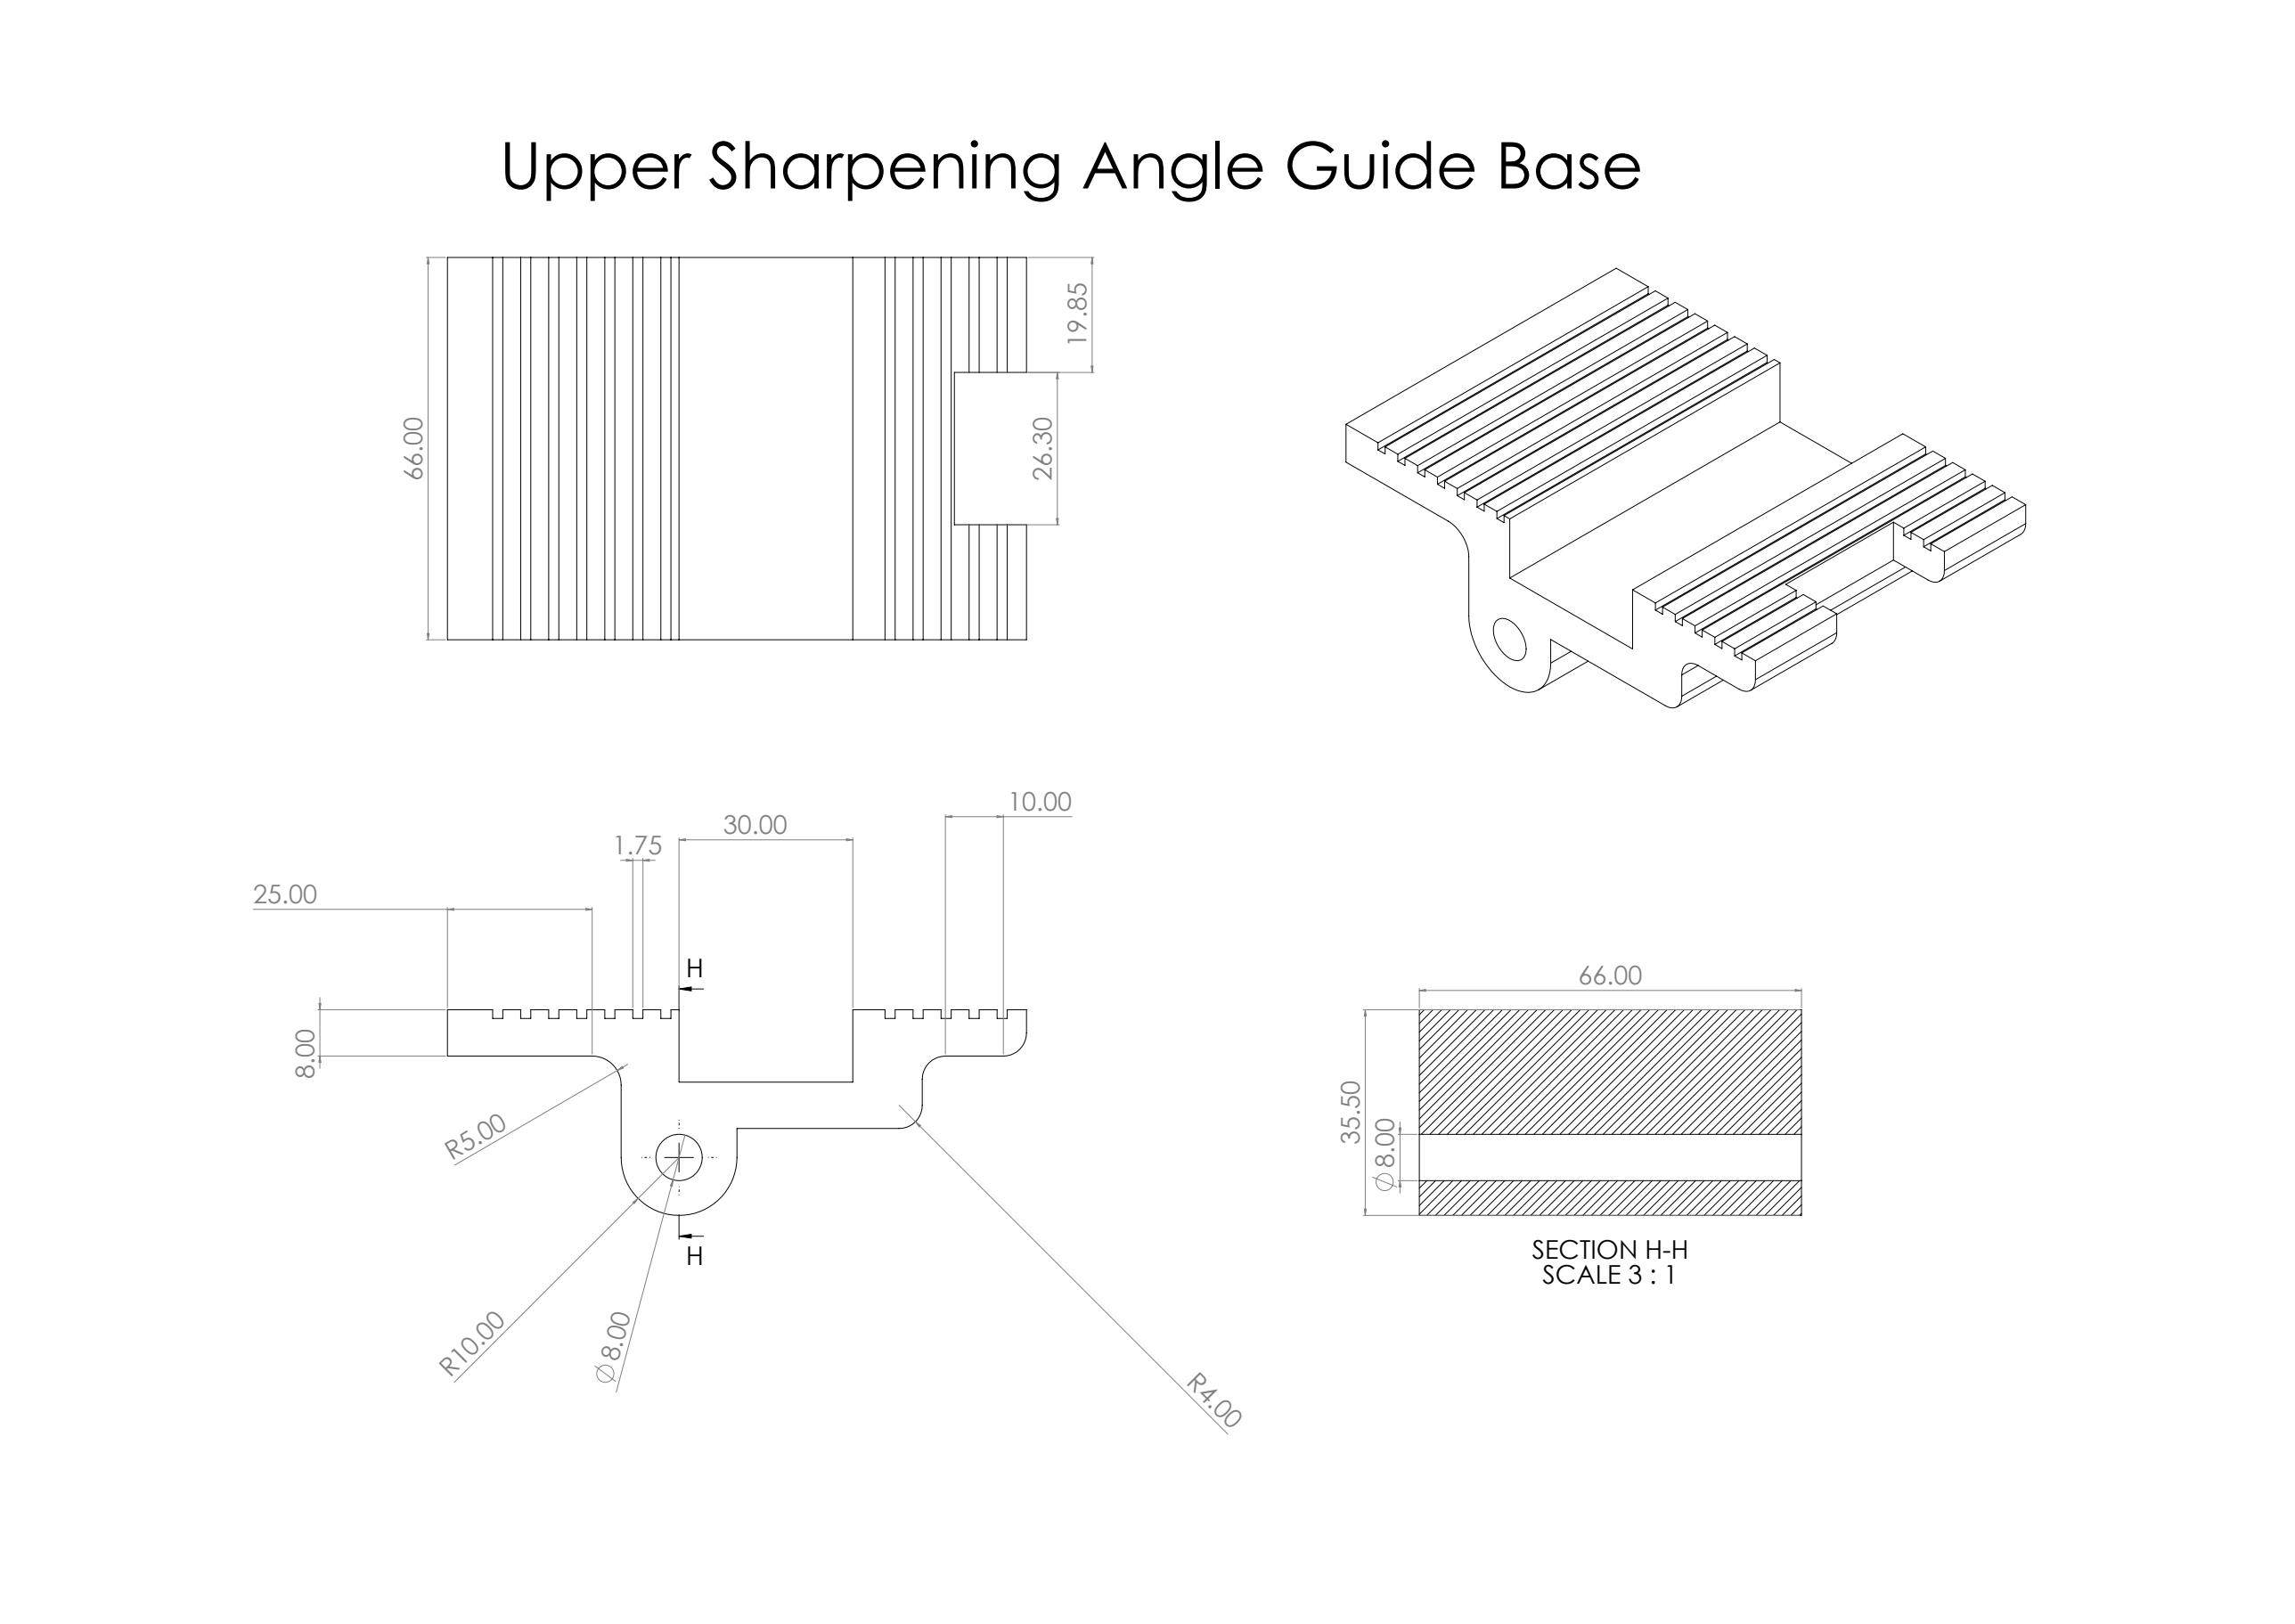
ISO-10303-21;
HEADER;
FILE_DESCRIPTION (('STEP AP214'),
    '1' );
FILE_NAME ('Upper Sharpening Angle Guide Base.step',
    '2026-10-24T21:31:31',
    ( '' ),
    ( '' ),
    'SwSTEP 2.0',
    'SolidWorks 2025',
    '' );
FILE_SCHEMA (( 'AUTOMOTIVE_DESIGN' ));
ENDSEC;

DATA;
#6=LINE ( 'NONE', #11694, #4610 ) ;
#13=LINE ( 'NONE', #7011, #3647 ) ;
#14=VECTOR ( 'NONE', #2004, 1000.000000000000000 ) ;
#17=DIRECTION ( 'NONE',  ( -1.000000000000000000, 0.000000000000000000, 0.000000000000000000 ) ) ;
#20=VERTEX_POINT ( 'NONE', #5429 ) ;
#32=FACE_OUTER_BOUND ( 'NONE', #11110, .T. ) ;
#33=ADVANCED_FACE ( 'NONE', ( #12199 ), #9834, .F. ) ;
#37=ORIENTED_EDGE ( 'NONE', *, *, #2232, .F. ) ;
#38=FACE_OUTER_BOUND ( 'NONE', #6545, .T. ) ;
#41=LINE ( 'NONE', #2497, #6085 ) ;
#42=AXIS2_PLACEMENT_3D ( 'NONE', #10885, #14351, #11948 ) ;
#47=CARTESIAN_POINT ( 'NONE',  ( 46.91810375148135392, 21.75070940071322667, 139.1143251403882459 ) ) ;
#49=CARTESIAN_POINT ( 'NONE',  ( -2.016677571526633510E-15, 23.25070940071368497, -33.00000000000012790 ) ) ;
#54=VECTOR ( 'NONE', #13573, 1000.000000000000000 ) ;
#57=LINE ( 'NONE', #11745, #6919 ) ;
#62=CARTESIAN_POINT ( 'NONE',  ( 114.6731053250840233, 21.75070940071369918, 139.1143251403882459 ) ) ;
#65=VERTEX_POINT ( 'NONE', #11047 ) ;
#66=VECTOR ( 'NONE', #7622, 1000.000000000000000 ) ;
#68=PLANE ( 'NONE',  #7695 ) ;
#72=VERTEX_POINT ( 'NONE', #721 ) ;
#75=PLANE ( 'NONE',  #1648 ) ;
#77=VERTEX_POINT ( 'NONE', #4338 ) ;
#86=VECTOR ( 'NONE', #1332, 1000.000000000000000 ) ;
#94=ORIENTED_EDGE ( 'NONE', *, *, #8937, .F. ) ;
#105=LINE ( 'NONE', #10640, #5976 ) ;
#108=DIRECTION ( 'NONE',  ( 0.000000000000000000, 0.000000000000000000, 1.000000000000000000 ) ) ;
#110=LINE ( 'NONE', #11941, #4147 ) ;
#114=ORIENTED_EDGE ( 'NONE', *, *, #14825, .F. ) ;
#116=CARTESIAN_POINT ( 'NONE',  ( 0.000000000000000000, 21.75070940071363168, 33.00000000000012790 ) ) ;
#118=LINE ( 'NONE', #8565, #1013 ) ;
#120=LINE ( 'NONE', #8431, #11123 ) ;
#130=ORIENTED_EDGE ( 'NONE', *, *, #11606, .T. ) ;
#132=ORIENTED_EDGE ( 'NONE', *, *, #1705, .F. ) ;
#133=DIRECTION ( 'NONE',  ( 1.000000000000000000, 0.000000000000000000, 0.000000000000000000 ) ) ;
#135=ORIENTED_EDGE ( 'NONE', *, *, #2741, .T. ) ;
#138=CARTESIAN_POINT ( 'NONE',  ( 48.00000000000000000, -2.249290599286307479, 139.1143251403882459 ) ) ;
#161=CARTESIAN_POINT ( 'NONE',  ( 42.07846078193830408, 21.75070940071319114, 139.1143251403882459 ) ) ;
#191=DIRECTION ( 'NONE',  ( 0.000000000000000000, 0.000000000000000000, 1.000000000000000000 ) ) ;
#197=DIRECTION ( 'NONE',  ( 1.000000000000000000, 0.000000000000000000, 0.000000000000000000 ) ) ;
#209=ORIENTED_EDGE ( 'NONE', *, *, #14302, .F. ) ;
#216=LINE ( 'NONE', #3742, #12117 ) ;
#218=PLANE ( 'NONE',  #1793 ) ;
#220=ORIENTED_EDGE ( 'NONE', *, *, #12965, .T. ) ;
#221=EDGE_LOOP ( 'NONE', ( #14150, #12830, #6180, #1820 ) ) ;
#222=EDGE_CURVE ( 'NONE', #13907, #15116, #14885, .T. ) ;
#235=LINE ( 'NONE', #14317, #9148 ) ;
#236=CARTESIAN_POINT ( 'NONE',  ( 118.0000000000000568, 2.046973701652633381E-13, 13.14990448602693007 ) ) ;
#240=CARTESIAN_POINT ( 'NONE',  ( 48.00000000000000711, 10.25070940071368497, -33.00000000000012790 ) ) ;
#249=CARTESIAN_POINT ( 'NONE',  ( 104.0000000000000426, 15.25070940071369563, -33.00000000000012790 ) ) ;
#254=FACE_OUTER_BOUND ( 'NONE', #221, .T. ) ;
#255=DIRECTION ( 'NONE',  ( 0.000000000000000000, 0.000000000000000000, -1.000000000000000000 ) ) ;
#257=DIRECTION ( 'NONE',  ( 0.000000000000000000, 1.000000000000000000, -0.000000000000000000 ) ) ;
#265=ORIENTED_EDGE ( 'NONE', *, *, #2651, .T. ) ;
#270=VECTOR ( 'NONE', #1744, 1000.000000000000000 ) ;
#273=DIRECTION ( 'NONE',  ( -0.000000000000000000, -0.000000000000000000, -1.000000000000000000 ) ) ;
#278=DIRECTION ( 'NONE',  ( 0.000000000000000000, 0.000000000000000000, -1.000000000000000000 ) ) ;
#291=VECTOR ( 'NONE', #10970, 1000.000000000000000 ) ;
#299=DIRECTION ( 'NONE',  ( 0.000000000000000000, 1.000000000000000000, 0.000000000000000000 ) ) ;
#315=PLANE ( 'NONE',  #10049 ) ;
#320=VECTOR ( 'NONE', #7998, 1000.000000000000000 ) ;
#321=ORIENTED_EDGE ( 'NONE', *, *, #14732, .T. ) ;
#322=VERTEX_POINT ( 'NONE', #10317 ) ;
#335=EDGE_CURVE ( 'NONE', #11258, #1446, #2933, .T. ) ;
#340=DIRECTION ( 'NONE',  ( 0.000000000000000000, 0.000000000000000000, 1.000000000000000000 ) ) ;
#344=VECTOR ( 'NONE', #582, 1000.000000000000000 ) ;
#351=EDGE_CURVE ( 'NONE', #1115, #11167, #14092, .T. ) ;
#352=CYLINDRICAL_SURFACE ( 'NONE', #8410, 4.000000000000003553 ) ;
#358=VERTEX_POINT ( 'NONE', #2315 ) ;
#359=DIRECTION ( 'NONE',  ( 1.000000000000000000, 0.000000000000000000, 0.000000000000000000 ) ) ;
#360=ORIENTED_EDGE ( 'NONE', *, *, #2072, .T. ) ;
#365=ORIENTED_EDGE ( 'NONE', *, *, #10647, .T. ) ;
#368=CARTESIAN_POINT ( 'NONE',  ( -2.688903428702175252E-15, 23.25070940071368142, 33.00000000000012790 ) ) ;
#370=CARTESIAN_POINT ( 'NONE',  ( 0.000000000000000000, 21.75070940071329417, 139.1143251403882459 ) ) ;
#380=ORIENTED_EDGE ( 'NONE', *, *, #7068, .T. ) ;
#387=EDGE_CURVE ( 'NONE', #550, #2283, #6562, .T. ) ;
#389=ORIENTED_EDGE ( 'NONE', *, *, #387, .F. ) ;
#391=ORIENTED_EDGE ( 'NONE', *, *, #15115, .F. ) ;
#398=CARTESIAN_POINT ( 'NONE',  ( 114.0000000000000284, 15.25070940071369563, 139.1143251403882459 ) ) ;
#402=AXIS2_PLACEMENT_3D ( 'NONE', #1965, #6663, #11352 ) ;
#411=FACE_OUTER_BOUND ( 'NONE', #3533, .T. ) ;
#417=( GEOMETRIC_REPRESENTATION_CONTEXT ( 3 ) GLOBAL_UNCERTAINTY_ASSIGNED_CONTEXT ( ( #1045 ) ) GLOBAL_UNIT_ASSIGNED_CONTEXT ( ( #9181, #13866, #10252 ) ) REPRESENTATION_CONTEXT ( 'NONE', 'WORKASPACE' ) );
#431=EDGE_CURVE ( 'NONE', #7143, #4346, #6, .T. ) ;
#449=EDGE_CURVE ( 'NONE', #4396, #5927, #2469, .T. ) ;
#456=EDGE_LOOP ( 'NONE', ( #15169, #3093, #13253, #6276 ) ) ;
#460=ORIENTED_EDGE ( 'NONE', *, *, #1519, .F. ) ;
#461=DIRECTION ( 'NONE',  ( -0.000000000000000000, -0.000000000000000000, -1.000000000000000000 ) ) ;
#481=PLANE ( 'NONE',  #13025 ) ;
#491=PLANE ( 'NONE',  #9839 ) ;
#514=DIRECTION ( 'NONE',  ( 0.000000000000000000, 1.000000000000000000, -0.000000000000000000 ) ) ;
#525=EDGE_CURVE ( 'NONE', #14965, #13020, #11921, .T. ) ;
#529=ORIENTED_EDGE ( 'NONE', *, *, #4885, .F. ) ;
#535=FACE_OUTER_BOUND ( 'NONE', #14760, .T. ) ;
#537=CARTESIAN_POINT ( 'NONE',  ( 114.6731053250840233, 0.000000000000000000, -33.00000000000012790 ) ) ;
#540=VECTOR ( 'NONE', #9041, 1000.000000000000000 ) ;
#541=CARTESIAN_POINT ( 'NONE',  ( 114.0000000000000284, 19.25070940071369563, 33.00000000000012790 ) ) ;
#542=VECTOR ( 'NONE', #2732, 1000.000000000000000 ) ;
#550=VERTEX_POINT ( 'NONE', #9855 ) ;
#558=AXIS2_PLACEMENT_3D ( 'NONE', #4944, #4869, #3708 ) ;
#560=VECTOR ( 'NONE', #4903, 1000.000000000000000 ) ;
#562=DIRECTION ( 'NONE',  ( -0.000000000000000000, -0.000000000000000000, -1.000000000000000000 ) ) ;
#565=ORIENTED_EDGE ( 'NONE', *, *, #14825, .T. ) ;
#571=LINE ( 'NONE', #6351, #6668 ) ;
#573=ADVANCED_FACE ( 'NONE', ( #1464 ), #315, .F. ) ;
#575=CARTESIAN_POINT ( 'NONE',  ( 95.31453344691183815, 23.25070940071369208, 33.00000000000012790 ) ) ;
#576=ORIENTED_EDGE ( 'NONE', *, *, #10446, .T. ) ;
#577=CARTESIAN_POINT ( 'NONE',  ( 0.000000000000000000, 15.25070940071369563, -13.14990448602693007 ) ) ;
#578=ORIENTED_EDGE ( 'NONE', *, *, #10333, .T. ) ;
#582=DIRECTION ( 'NONE',  ( 0.000000000000000000, 1.000000000000000000, -0.000000000000000000 ) ) ;
#584=ORIENTED_EDGE ( 'NONE', *, *, #12621, .T. ) ;
#587=VERTEX_POINT ( 'NONE', #10936 ) ;
#588=DIRECTION ( 'NONE',  ( -1.000000000000000000, 0.000000000000000000, 0.000000000000000000 ) ) ;
#589=ORIENTED_EDGE ( 'NONE', *, *, #1386, .T. ) ;
#600=CARTESIAN_POINT ( 'NONE',  ( 32.39917484285220439, 21.75070940071312364, 33.00000000000012790 ) ) ;
#613=LINE ( 'NONE', #1772, #10037 ) ;
#620=DIRECTION ( 'NONE',  ( -1.000000000000000000, 0.000000000000000000, 0.000000000000000000 ) ) ;
#626=CARTESIAN_POINT ( 'NONE',  ( 45.17127246049422240, 21.75070940071322667, 139.1143251403882459 ) ) ;
#628=CARTESIAN_POINT ( 'NONE',  ( 43.00000000000000711, 15.25070940071368497, 33.00000000000012790 ) ) ;
#637=CARTESIAN_POINT ( 'NONE',  ( 0.000000000000000000, 15.25070940071369563, 13.14990448602693007 ) ) ;
#642=DIRECTION ( 'NONE',  ( 0.000000000000000000, 0.000000000000000000, 1.000000000000000000 ) ) ;
#647=EDGE_CURVE ( 'NONE', #13534, #13054, #13162, .T. ) ;
#648=LINE ( 'NONE', #5356, #9186 ) ;
#659=CARTESIAN_POINT ( 'NONE',  ( 27.55953187330915810, 23.25070940071368852, -33.00000000000012790 ) ) ;
#660=CARTESIAN_POINT ( 'NONE',  ( 0.000000000000000000, 15.25070940071368497, 139.1143251403882459 ) ) ;
#661=LINE ( 'NONE', #891, #6723 ) ;
#665=VECTOR ( 'NONE', #12241, 1000.000000000000000 ) ;
#675=PRODUCT ( 'Upper Sharpening Angle Guide Base', 'Upper Sharpening Angle Guide Base', '', ( #1396 ) ) ;
#678=ORIENTED_EDGE ( 'NONE', *, *, #2260, .T. ) ;
#686=CARTESIAN_POINT ( 'NONE',  ( 18.00000000000001066, 0.000000000000000000, 139.1143251403882459 ) ) ;
#696=CARTESIAN_POINT ( 'NONE',  ( 25.81270058232203013, 21.75070940071309167, -33.00000000000012790 ) ) ;
#703=AXIS2_PLACEMENT_3D ( 'NONE', #8419, #1403, #8107 ) ;
#719=AXIS2_PLACEMENT_3D ( 'NONE', #5968, #10655, #14038 ) ;
#721=CARTESIAN_POINT ( 'NONE',  ( 114.0000000000000284, 15.25070940071369563, -13.14990448602693007 ) ) ;
#729=ORIENTED_EDGE ( 'NONE', *, *, #11145, .F. ) ;
#731=ORIENTED_EDGE ( 'NONE', *, *, #3102, .F. ) ;
#735=CARTESIAN_POINT ( 'NONE',  ( 68.00000000000001421, -2.249290599286293268, 33.00000000000012790 ) ) ;
#738=DIRECTION ( 'NONE',  ( 1.110223024625156540E-15, -1.000000000000000000, 0.000000000000000000 ) ) ;
#741=ADVANCED_FACE ( 'NONE', ( #11639 ), #15109, .F. ) ;
#745=ORIENTED_EDGE ( 'NONE', *, *, #13734, .T. ) ;
#749=ORIENTED_EDGE ( 'NONE', *, *, #11198, .T. ) ;
#751=ADVANCED_FACE ( 'NONE', ( #11790, #1325 ), #12724, .F. ) ;
#757=DIRECTION ( 'NONE',  ( -2.775557561562891351E-15, 1.000000000000000000, 0.000000000000000000 ) ) ;
#766=ORIENTED_EDGE ( 'NONE', *, *, #5761, .T. ) ;
#767=VECTOR ( 'NONE', #133, 1000.000000000000000 ) ;
#778=CARTESIAN_POINT ( 'NONE',  ( 118.0000000000000284, 23.25070940071369563, 139.1143251403882459 ) ) ;
#782=CARTESIAN_POINT ( 'NONE',  ( 30.65234355186507997, 21.75070940071312364, 139.1143251403882459 ) ) ;
#794=ORIENTED_EDGE ( 'NONE', *, *, #3873, .F. ) ;
#799=ADVANCED_FACE ( 'NONE', ( #1173 ), #14109, .F. ) ;
#804=CARTESIAN_POINT ( 'NONE',  ( 51.75774672102440377, 21.75070940071325865, -33.00000000000012790 ) ) ;
#809=ORIENTED_EDGE ( 'NONE', *, *, #5886, .F. ) ;
#812=CARTESIAN_POINT ( 'NONE',  ( 103.2469880950108063, 23.25070940071369208, -33.00000000000012790 ) ) ;
#813=LINE ( 'NONE', #2986, #1383 ) ;
#815=CARTESIAN_POINT ( 'NONE',  ( 46.91810375148135392, 23.25070940071368852, 33.00000000000012790 ) ) ;
#826=ORIENTED_EDGE ( 'NONE', *, *, #11805, .F. ) ;
#830=CARTESIAN_POINT ( 'NONE',  ( 100.0000000000000284, 11.25070940071369563, -33.00000000000012790 ) ) ;
#836=FACE_OUTER_BOUND ( 'NONE', #10102, .T. ) ;
#837=ADVANCED_FACE ( 'NONE', ( #8103 ), #14260, .F. ) ;
#838=ORIENTED_EDGE ( 'NONE', *, *, #12621, .F. ) ;
#844=VERTEX_POINT ( 'NONE', #5167 ) ;
#845=ADVANCED_FACE ( 'NONE', ( #1698 ), #6393, .F. ) ;
#847=LINE ( 'NONE', #1850, #4677 ) ;
#850=DIRECTION ( 'NONE',  ( 1.000000000000000000, 1.156482317317870492E-16, 0.000000000000000000 ) ) ;
#855=LINE ( 'NONE', #14787, #8320 ) ;
#857=APPLICATION_CONTEXT ( 'automotive_design' ) ;
#862=FACE_OUTER_BOUND ( 'NONE', #2285, .T. ) ;
#868=ORIENTED_EDGE ( 'NONE', *, *, #13611, .F. ) ;
#869=CARTESIAN_POINT ( 'NONE',  ( 30.65234355186507997, 23.25070940071368852, 33.00000000000012790 ) ) ;
#871=ORIENTED_EDGE ( 'NONE', *, *, #15074, .F. ) ;
#874=AXIS2_PLACEMENT_3D ( 'NONE', #14984, #10447, #6820 ) ;
#891=CARTESIAN_POINT ( 'NONE',  ( -2.016677571526633510E-15, 23.25070940071368497, 33.00000000000012790 ) ) ;
#906=EDGE_LOOP ( 'NONE', ( #132, #13235, #5815, #2969 ) ) ;
#914=CARTESIAN_POINT ( 'NONE',  ( 109.8334623555409735, 0.000000000000000000, 13.14990448602693007 ) ) ;
#916=VECTOR ( 'NONE', #1039, 1000.000000000000000 ) ;
#925=DIRECTION ( 'NONE',  ( 0.000000000000000000, 1.000000000000000000, 0.000000000000000000 ) ) ;
#930=CARTESIAN_POINT ( 'NONE',  ( 112.9262740340969060, 0.000000000000000000, 139.1143251403882459 ) ) ;
#937=EDGE_CURVE ( 'NONE', #7143, #11623, #10072, .T. ) ;
#941=CARTESIAN_POINT ( 'NONE',  ( 0.000000000000000000, 21.75070940071325865, 139.1143251403882459 ) ) ;
#957=CARTESIAN_POINT ( 'NONE',  ( 40.33162949095117966, 23.25070940071368852, -33.00000000000012790 ) ) ;
#970=AXIS2_PLACEMENT_3D ( 'NONE', #941, #13800, #11326 ) ;
#973=DIRECTION ( 'NONE',  ( 1.000000000000000000, 1.156482317317870492E-16, 0.000000000000000000 ) ) ;
#977=VERTEX_POINT ( 'NONE', #14993 ) ;
#980=CARTESIAN_POINT ( 'NONE',  ( -2.688903428702175252E-15, 23.25070940071368142, 33.00000000000012790 ) ) ;
#982=AXIS2_PLACEMENT_3D ( 'NONE', #8563, #2856, #340 ) ;
#992=CARTESIAN_POINT ( 'NONE',  ( 0.000000000000000000, 21.75070940071309167, 139.1143251403882459 ) ) ;
#1003=ORIENTED_EDGE ( 'NONE', *, *, #8126, .F. ) ;
#1007=DIRECTION ( 'NONE',  ( -0.000000000000000000, -0.000000000000000000, -1.000000000000000000 ) ) ;
#1012=DIRECTION ( 'NONE',  ( -0.000000000000000000, 0.000000000000000000, 1.000000000000000000 ) ) ;
#1013=VECTOR ( 'NONE', #13265, 1000.000000000000000 ) ;
#1035=LINE ( 'NONE', #2428, #12248 ) ;
#1037=CARTESIAN_POINT ( 'NONE',  ( 27.55953187330915810, 21.75070940071309167, 139.1143251403882459 ) ) ;
#1039=DIRECTION ( 'NONE',  ( -1.000000000000000000, -1.156482317317870492E-16, 0.000000000000000000 ) ) ;
#1045=UNCERTAINTY_MEASURE_WITH_UNIT (LENGTH_MEASURE( 1.000000000000000082E-05 ), #9181, 'distance_accuracy_value', 'NONE');
#1047=ORIENTED_EDGE ( 'NONE', *, *, #11121, .T. ) ;
#1053=ADVANCED_FACE ( 'NONE', ( #1060 ), #68, .F. ) ;
#1054=CARTESIAN_POINT ( 'NONE',  ( 45.17127246049422240, 21.75070940071322667, 33.00000000000012790 ) ) ;
#1060=FACE_OUTER_BOUND ( 'NONE', #4938, .T. ) ;
#1074=DIRECTION ( 'NONE',  ( 0.000000000000000000, 1.000000000000000000, -0.000000000000000000 ) ) ;
#1091=CARTESIAN_POINT ( 'NONE',  ( -2.688903428702175252E-15, 23.25070940071368142, 139.1143251403882459 ) ) ;
#1104=DIRECTION ( 'NONE',  ( 0.000000000000000000, 1.000000000000000000, 0.000000000000000000 ) ) ;
#1110=LINE ( 'NONE', #2350, #5012 ) ;
#1115=VERTEX_POINT ( 'NONE', #10454 ) ;
#1117=VERTEX_POINT ( 'NONE', #9537 ) ;
#1120=DIRECTION ( 'NONE',  ( -1.000000000000000000, 0.000000000000000000, 0.000000000000000000 ) ) ;
#1121=VECTOR ( 'NONE', #11160, 1000.000000000000000 ) ;
#1127=CARTESIAN_POINT ( 'NONE',  ( 50.01091543003727224, 0.000000000000000000, -33.00000000000012790 ) ) ;
#1132=ORIENTED_EDGE ( 'NONE', *, *, #2690, .T. ) ;
#1137=ORIENTED_EDGE ( 'NONE', *, *, #10778, .F. ) ;
#1143=EDGE_CURVE ( 'NONE', #6567, #14796, #12851, .T. ) ;
#1144=AXIS2_PLACEMENT_3D ( 'NONE', #660, #5528, #12372 ) ;
#1146=DIRECTION ( 'NONE',  ( 1.000000000000000000, -0.000000000000000000, -0.000000000000000000 ) ) ;
#1150=DIRECTION ( 'NONE',  ( 1.734723475976807292E-15, -1.000000000000000000, 0.000000000000000000 ) ) ;
#1151=CARTESIAN_POINT ( 'NONE',  ( 54.00000000000000711, -2.249290599286311032, 33.00000000000012790 ) ) ;
#1153=ADVANCED_FACE ( 'NONE', ( #11515 ), #2215, .F. ) ;
#1173=FACE_OUTER_BOUND ( 'NONE', #9518, .T. ) ;
#1175=EDGE_CURVE ( 'NONE', #10461, #3922, #7367, .T. ) ;
#1176=VECTOR ( 'NONE', #14022, 1000.000000000000000 ) ;
#1178=FACE_OUTER_BOUND ( 'NONE', #3126, .T. ) ;
#1189=VECTOR ( 'NONE', #10286, 1000.000000000000000 ) ;
#1190=EDGE_LOOP ( 'NONE', ( #8131, #3911, #5540, #4860 ) ) ;
#1205=ORIENTED_EDGE ( 'NONE', *, *, #6548, .T. ) ;
#1216=ORIENTED_EDGE ( 'NONE', *, *, #4415, .T. ) ;
#1222=EDGE_CURVE ( 'NONE', #20, #13907, #11903, .T. ) ;
#1225=EDGE_LOOP ( 'NONE', ( #8488, #1205, #7597, #4474 ) ) ;
#1231=DIRECTION ( 'NONE',  ( 1.000000000000000000, 0.000000000000000000, 0.000000000000000000 ) ) ;
#1239=DIRECTION ( 'NONE',  ( -1.110223024625156540E-15, 1.000000000000000000, 0.000000000000000000 ) ) ;
#1254=VECTOR ( 'NONE', #14887, 1000.000000000000000 ) ;
#1256=ORIENTED_EDGE ( 'NONE', *, *, #1813, .F. ) ;
#1257=DIRECTION ( 'NONE',  ( 0.000000000000000000, 0.000000000000000000, 1.000000000000000000 ) ) ;
#1261=ADVANCED_FACE ( 'NONE', ( #9762 ), #6148, .T. ) ;
#1262=CARTESIAN_POINT ( 'NONE',  ( -1.243300532054838308E-15, 10.75070940071368142, -33.00000000000012790 ) ) ;
#1263=VECTOR ( 'NONE', #5764, 1000.000000000000000 ) ;
#1275=LINE ( 'NONE', #10675, #767 ) ;
#1280=ADVANCED_FACE ( 'NONE', ( #8522, #10758 ), #218, .T. ) ;
#1288=AXIS2_PLACEMENT_3D ( 'NONE', #12935, #13082, #1377 ) ;
#1289=EDGE_LOOP ( 'NONE', ( #2796, #13787, #11153, #13533, #11758, #578, #321, #745 ) ) ;
#1297=VECTOR ( 'NONE', #3657, 1000.000000000000000 ) ;
#1300=CARTESIAN_POINT ( 'NONE',  ( -2.688903428702175252E-15, 23.25070940071368142, 33.00000000000012790 ) ) ;
#1308=DIRECTION ( 'NONE',  ( -0.000000000000000000, -0.000000000000000000, -1.000000000000000000 ) ) ;
#1312=VECTOR ( 'NONE', #7448, 1000.000000000000000 ) ;
#1324=LINE ( 'NONE', #11711, #12676 ) ;
#1325=FACE_BOUND ( 'NONE', #10555, .T. ) ;
#1332=DIRECTION ( 'NONE',  ( -1.000000000000000000, -8.673617379884035472E-17, 0.000000000000000000 ) ) ;
#1346=EDGE_CURVE ( 'NONE', #358, #13613, #648, .T. ) ;
#1352=DIRECTION ( 'NONE',  ( 0.000000000000000000, 1.000000000000000000, -0.000000000000000000 ) ) ;
#1355=DIRECTION ( 'NONE',  ( 0.000000000000000000, 1.000000000000000000, -0.000000000000000000 ) ) ;
#1361=EDGE_CURVE ( 'NONE', #6460, #12669, #7742, .T. ) ;
#1364=EDGE_CURVE ( 'NONE', #11647, #12323, #3195, .T. ) ;
#1367=ORIENTED_EDGE ( 'NONE', *, *, #15114, .T. ) ;
#1377=DIRECTION ( 'NONE',  ( 0.000000000000000000, 0.000000000000000000, 1.000000000000000000 ) ) ;
#1379=DIRECTION ( 'NONE',  ( 0.000000000000000000, -1.000000000000000000, 0.000000000000000000 ) ) ;
#1381=EDGE_LOOP ( 'NONE', ( #15083, #10267, #135, #6493 ) ) ;
#1382=EDGE_CURVE ( 'NONE', #13652, #4131, #6504, .T. ) ;
#1383=VECTOR ( 'NONE', #1822, 1000.000000000000000 ) ;
#1385=LINE ( 'NONE', #5078, #7650 ) ;
#1386=EDGE_CURVE ( 'NONE', #5719, #5462, #7705, .T. ) ;
#1391=ORIENTED_EDGE ( 'NONE', *, *, #13173, .T. ) ;
#1394=ORIENTED_EDGE ( 'NONE', *, *, #6976, .F. ) ;
#1396=PRODUCT_CONTEXT ( 'NONE', #857, 'mechanical' ) ;
#1397=DIRECTION ( 'NONE',  ( 1.000000000000000000, 1.156482317317870492E-16, 0.000000000000000000 ) ) ;
#1398=DIRECTION ( 'NONE',  ( 0.000000000000000000, 1.000000000000000000, -0.000000000000000000 ) ) ;
#1401=VECTOR ( 'NONE', #6292, 1000.000000000000000 ) ;
#1403=DIRECTION ( 'NONE',  ( 0.000000000000000000, 0.000000000000000000, -1.000000000000000000 ) ) ;
#1414=CARTESIAN_POINT ( 'NONE',  ( 35.49198652140812982, 23.25070940071368852, -33.00000000000012790 ) ) ;
#1426=ORIENTED_EDGE ( 'NONE', *, *, #10139, .F. ) ;
#1438=CARTESIAN_POINT ( 'NONE',  ( 58.00000000000000711, 0.000000000000000000, 33.00000000000012790 ) ) ;
#1444=LINE ( 'NONE', #4764, #6559 ) ;
#1445=ORIENTED_EDGE ( 'NONE', *, *, #12870, .T. ) ;
#1446=VERTEX_POINT ( 'NONE', #7822 ) ;
#1448=ORIENTED_EDGE ( 'NONE', *, *, #8487, .F. ) ;
#1457=EDGE_CURVE ( 'NONE', #3968, #9234, #11416, .T. ) ;
#1460=VERTEX_POINT ( 'NONE', #804 ) ;
#1464=FACE_OUTER_BOUND ( 'NONE', #14437, .T. ) ;
#1467=ORIENTED_EDGE ( 'NONE', *, *, #4385, .F. ) ;
#1472=CARTESIAN_POINT ( 'NONE',  ( 54.85055839958032209, 21.75070940071329417, -33.00000000000012790 ) ) ;
#1501=AXIS2_PLACEMENT_3D ( 'NONE', #5150, #14538, #4054 ) ;
#1506=VERTEX_POINT ( 'NONE', #8049 ) ;
#1510=AXIS2_PLACEMENT_3D ( 'NONE', #4667, #12835, #13133 ) ;
#1511=CARTESIAN_POINT ( 'NONE',  ( 35.49198652140812982, 21.75070940071315562, -33.00000000000012790 ) ) ;
#1519=EDGE_CURVE ( 'NONE', #14965, #977, #1110, .T. ) ;
#1524=EDGE_LOOP ( 'NONE', ( #11746, #12539, #5464, #7230 ) ) ;
#1527=VERTEX_POINT ( 'NONE', #957 ) ;
#1529=EDGE_CURVE ( 'NONE', #4620, #12466, #3431, .T. ) ;
#1537=ORIENTED_EDGE ( 'NONE', *, *, #6853, .F. ) ;
#1549=VERTEX_POINT ( 'NONE', #10515 ) ;
#1551=VECTOR ( 'NONE', #10800, 1000.000000000000000 ) ;
#1555=CARTESIAN_POINT ( 'NONE',  ( 0.000000000000000000, 21.75070940071369918, -33.00000000000012790 ) ) ;
#1556=LINE ( 'NONE', #5543, #8188 ) ;
#1559=ORIENTED_EDGE ( 'NONE', *, *, #10247, .T. ) ;
#1567=EDGE_CURVE ( 'NONE', #3404, #4646, #2275, .T. ) ;
#1570=CARTESIAN_POINT ( 'NONE',  ( 30.65234355186507997, 21.75070940071312364, -33.00000000000012790 ) ) ;
#1581=CARTESIAN_POINT ( 'NONE',  ( 112.9262740340969060, 0.000000000000000000, -33.00000000000012790 ) ) ;
#1583=CARTESIAN_POINT ( 'NONE',  ( 18.00000000000001066, 0.000000000000000000, -33.00000000000012790 ) ) ;
#1593=CARTESIAN_POINT ( 'NONE',  ( 112.9262740340969060, 0.000000000000000000, 33.00000000000012790 ) ) ;
#1614=CARTESIAN_POINT ( 'NONE',  ( 114.6731053250840233, 23.25070940071369563, 139.1143251403882459 ) ) ;
#1629=DIRECTION ( 'NONE',  ( -0.000000000000000000, -0.000000000000000000, 1.000000000000000000 ) ) ;
#1632=VECTOR ( 'NONE', #13443, 1000.000000000000000 ) ;
#1648=AXIS2_PLACEMENT_3D ( 'NONE', #11908, #9701, #13294 ) ;
#1650=DIRECTION ( 'NONE',  ( 0.000000000000000000, 1.000000000000000000, -0.000000000000000000 ) ) ;
#1670=DIRECTION ( 'NONE',  ( 0.000000000000000000, 1.000000000000000000, -0.000000000000000000 ) ) ;
#1672=ORIENTED_EDGE ( 'NONE', *, *, #10963, .F. ) ;
#1674=ORIENTED_EDGE ( 'NONE', *, *, #3328, .F. ) ;
#1679=VERTEX_POINT ( 'NONE', #8025 ) ;
#1682=CARTESIAN_POINT ( 'NONE',  ( 105.5545870572953930, 15.25070940071369563, -13.14990448602692474 ) ) ;
#1691=VERTEX_POINT ( 'NONE', #3410 ) ;
#1692=ORIENTED_EDGE ( 'NONE', *, *, #11765, .T. ) ;
#1697=DIRECTION ( 'NONE',  ( 0.000000000000000000, 1.000000000000000000, -0.000000000000000000 ) ) ;
#1698=FACE_OUTER_BOUND ( 'NONE', #8312, .T. ) ;
#1705=EDGE_CURVE ( 'NONE', #20, #9290, #6865, .T. ) ;
#1707=FACE_OUTER_BOUND ( 'NONE', #14370, .T. ) ;
#1721=EDGE_CURVE ( 'NONE', #13543, #1911, #5496, .T. ) ;
#1733=DIRECTION ( 'NONE',  ( -0.000000000000000000, -0.000000000000000000, -1.000000000000000000 ) ) ;
#1744=DIRECTION ( 'NONE',  ( 0.000000000000000000, 1.000000000000000000, -0.000000000000000000 ) ) ;
#1757=DIRECTION ( 'NONE',  ( -0.000000000000000000, -0.000000000000000000, -1.000000000000000000 ) ) ;
#1760=FACE_OUTER_BOUND ( 'NONE', #8836, .T. ) ;
#1772=CARTESIAN_POINT ( 'NONE',  ( 54.00000000000000711, -2.249290599286311032, 139.1143251403882459 ) ) ;
#1773=AXIS2_PLACEMENT_3D ( 'NONE', #8136, #7618, #11156 ) ;
#1779=ORIENTED_EDGE ( 'NONE', *, *, #6089, .F. ) ;
#1788=VERTEX_POINT ( 'NONE', #8494 ) ;
#1790=EDGE_CURVE ( 'NONE', #8955, #2597, #4873, .T. ) ;
#1793=AXIS2_PLACEMENT_3D ( 'NONE', #6361, #13067, #12201 ) ;
#1807=LINE ( 'NONE', #637, #3513 ) ;
#1809=VERTEX_POINT ( 'NONE', #4945 ) ;
#1813=EDGE_CURVE ( 'NONE', #9234, #13543, #6111, .T. ) ;
#1820=ORIENTED_EDGE ( 'NONE', *, *, #3813, .F. ) ;
#1822=DIRECTION ( 'NONE',  ( -0.000000000000000000, -0.000000000000000000, -1.000000000000000000 ) ) ;
#1830=ADVANCED_FACE ( 'NONE', ( #8267 ), #6033, .T. ) ;
#1833=DIRECTION ( 'NONE',  ( 0.000000000000000000, 1.000000000000000000, -0.000000000000000000 ) ) ;
#1834=VERTEX_POINT ( 'NONE', #9654 ) ;
#1838=VERTEX_POINT ( 'NONE', #13180 ) ;
#1841=ADVANCED_FACE ( 'NONE', ( #1178 ), #14413, .T. ) ;
#1844=VERTEX_POINT ( 'NONE', #10571 ) ;
#1846=CARTESIAN_POINT ( 'NONE',  ( 45.17127246049422240, 0.000000000000000000, 33.00000000000012790 ) ) ;
#1848=ORIENTED_EDGE ( 'NONE', *, *, #2501, .F. ) ;
#1850=CARTESIAN_POINT ( 'NONE',  ( 95.31453344691183815, 23.25070940071369208, 139.1143251403882459 ) ) ;
#1860=PLANE ( 'NONE',  #8128 ) ;
#1866=DIRECTION ( 'NONE',  ( 1.156482317317871725E-16, -1.000000000000000000, 0.000000000000000000 ) ) ;
#1872=EDGE_CURVE ( 'NONE', #1691, #14241, #5960, .T. ) ;
#1883=EDGE_CURVE ( 'NONE', #7515, #2307, #5845, .T. ) ;
#1893=CARTESIAN_POINT ( 'NONE',  ( 35.49198652140812982, 0.000000000000000000, 139.1143251403882459 ) ) ;
#1905=VERTEX_POINT ( 'NONE', #3048 ) ;
#1907=VERTEX_POINT ( 'NONE', #7892 ) ;
#1908=CARTESIAN_POINT ( 'NONE',  ( 42.07846078193830408, 23.25070940071368852, -33.00000000000012790 ) ) ;
#1911=VERTEX_POINT ( 'NONE', #4339 ) ;
#1920=DIRECTION ( 'NONE',  ( -2.775557561562891351E-15, 1.000000000000000000, 0.000000000000000000 ) ) ;
#1924=ORIENTED_EDGE ( 'NONE', *, *, #3689, .F. ) ;
#1926=CARTESIAN_POINT ( 'NONE',  ( 54.85055839958032209, 0.000000000000000000, 139.1143251403882459 ) ) ;
#1927=ORIENTED_EDGE ( 'NONE', *, *, #12887, .F. ) ;
#1932=CARTESIAN_POINT ( 'NONE',  ( 112.9262740340969060, 23.25070940071369563, 139.1143251403882459 ) ) ;
#1938=AXIS2_PLACEMENT_3D ( 'NONE', #13715, #5489, #850 ) ;
#1948=DIRECTION ( 'NONE',  ( -1.000000000000000000, 0.000000000000000000, 0.000000000000000000 ) ) ;
#1956=DIRECTION ( 'NONE',  ( 0.000000000000000000, -1.000000000000000000, 0.000000000000000000 ) ) ;
#1958=VECTOR ( 'NONE', #6701, 1000.000000000000000 ) ;
#1965=CARTESIAN_POINT ( 'NONE',  ( 51.75774672102440377, 0.000000000000000000, 139.1143251403882459 ) ) ;
#1972=ORIENTED_EDGE ( 'NONE', *, *, #7774, .T. ) ;
#1983=CARTESIAN_POINT ( 'NONE',  ( 98.40734512546775647, 23.25070940071369208, -33.00000000000012790 ) ) ;
#1996=CARTESIAN_POINT ( 'NONE',  ( 108.0866310645538562, 23.25070940071369563, 33.00000000000012790 ) ) ;
#2004=DIRECTION ( 'NONE',  ( 0.000000000000000000, 1.000000000000000000, -0.000000000000000000 ) ) ;
#2005=EDGE_LOOP ( 'NONE', ( #13844, #10093, #5618, #6415 ) ) ;
#2009=FACE_OUTER_BOUND ( 'NONE', #13278, .T. ) ;
#2019=EDGE_CURVE ( 'NONE', #8234, #7396, #8440, .T. ) ;
#2029=LINE ( 'NONE', #6722, #8175 ) ;
#2031=CARTESIAN_POINT ( 'NONE',  ( 50.01091543003727224, 0.000000000000000000, 33.00000000000012790 ) ) ;
#2042=VECTOR ( 'NONE', #13527, 1000.000000000000000 ) ;
#2044=DIRECTION ( 'NONE',  ( 0.000000000000000000, 0.000000000000000000, -1.000000000000000000 ) ) ;
#2045=AXIS2_PLACEMENT_3D ( 'NONE', #2916, #4283, #8985 ) ;
#2055=ORIENTED_EDGE ( 'NONE', *, *, #13611, .T. ) ;
#2066=LINE ( 'NONE', #14079, #8795 ) ;
#2072=EDGE_CURVE ( 'NONE', #844, #13652, #11497, .T. ) ;
#2073=CARTESIAN_POINT ( 'NONE',  ( 114.6731053250840233, 21.75070940071369918, 139.1143251403882459 ) ) ;
#2083=EDGE_CURVE ( 'NONE', #12669, #3922, #4810, .T. ) ;
#2084=LINE ( 'NONE', #12556, #14 ) ;
#2086=CARTESIAN_POINT ( 'NONE',  ( 130.4454129427046496, 23.25070940071369563, -13.14990448602692474 ) ) ;
#2090=ORIENTED_EDGE ( 'NONE', *, *, #525, .T. ) ;
#2096=ORIENTED_EDGE ( 'NONE', *, *, #9756, .F. ) ;
#2097=ORIENTED_EDGE ( 'NONE', *, *, #7253, .F. ) ;
#2099=CARTESIAN_POINT ( 'NONE',  ( 112.9262740340969060, 21.75070940071369918, 33.00000000000012790 ) ) ;
#2117=EDGE_LOOP ( 'NONE', ( #3377, #9705, #678, #7452 ) ) ;
#2119=VECTOR ( 'NONE', #2226, 1000.000000000000000 ) ;
#2120=ORIENTED_EDGE ( 'NONE', *, *, #8390, .T. ) ;
#2122=VECTOR ( 'NONE', #7507, 1000.000000000000000 ) ;
#2123=EDGE_CURVE ( 'NONE', #8184, #7261, #9511, .T. ) ;
#2124=FACE_OUTER_BOUND ( 'NONE', #9570, .T. ) ;
#2134=CARTESIAN_POINT ( 'NONE',  ( 62.00000000000001421, -2.249290599286310588, 139.1143251403882459 ) ) ;
#2144=EDGE_CURVE ( 'NONE', #1115, #5061, #1035, .T. ) ;
#2148=DIRECTION ( 'NONE',  ( -0.000000000000000000, -0.000000000000000000, -1.000000000000000000 ) ) ;
#2149=CARTESIAN_POINT ( 'NONE',  ( 103.2469880950108063, 23.25070940071369208, 33.00000000000012790 ) ) ;
#2150=ORIENTED_EDGE ( 'NONE', *, *, #3689, .T. ) ;
#2157=AXIS2_PLACEMENT_3D ( 'NONE', #2634, #7329, #9578 ) ;
#2165=DIRECTION ( 'NONE',  ( 0.000000000000000000, -0.000000000000000000, 1.000000000000000000 ) ) ;
#2167=EDGE_LOOP ( 'NONE', ( #2376, #14738, #11687, #7222 ) ) ;
#2174=EDGE_CURVE ( 'NONE', #8402, #322, #15127, .T. ) ;
#2178=DIRECTION ( 'NONE',  ( -0.000000000000000000, -0.000000000000000000, -1.000000000000000000 ) ) ;
#2189=ORIENTED_EDGE ( 'NONE', *, *, #8041, .T. ) ;
#2191=CARTESIAN_POINT ( 'NONE',  ( 37.23881781239525424, 21.75070940071315562, 139.1143251403882459 ) ) ;
#2197=CARTESIAN_POINT ( 'NONE',  ( 105.5545870572953930, -1.749290599286305259, 13.14990448602692474 ) ) ;
#2201=ORIENTED_EDGE ( 'NONE', *, *, #14114, .F. ) ;
#2203=ORIENTED_EDGE ( 'NONE', *, *, #9582, .F. ) ;
#2210=PLANE ( 'NONE',  #874 ) ;
#2215=PLANE ( 'NONE',  #10403 ) ;
#2216=ADVANCED_FACE ( 'NONE', ( #13199 ), #4069, .F. ) ;
#2226=DIRECTION ( 'NONE',  ( -1.000000000000000000, -1.156482317317870492E-16, 0.000000000000000000 ) ) ;
#2227=PLANE ( 'NONE',  #7931 ) ;
#2231=ORIENTED_EDGE ( 'NONE', *, *, #2415, .T. ) ;
#2232=EDGE_CURVE ( 'NONE', #2283, #1907, #613, .T. ) ;
#2236=CARTESIAN_POINT ( 'NONE',  ( 48.00000000000000000, -2.664535259100377906E-14, 33.00000000000012790 ) ) ;
#2241=DIRECTION ( 'NONE',  ( -5.551115123125787632E-16, -1.000000000000000000, 0.000000000000000000 ) ) ;
#2252=CARTESIAN_POINT ( 'NONE',  ( 35.49198652140812982, 23.25070940071368852, 33.00000000000012790 ) ) ;
#2259=ORIENTED_EDGE ( 'NONE', *, *, #3210, .F. ) ;
#2260=EDGE_CURVE ( 'NONE', #8536, #12694, #13705, .T. ) ;
#2261=CARTESIAN_POINT ( 'NONE',  ( -2.688903428702175252E-15, 23.25070940071368142, 139.1143251403882459 ) ) ;
#2265=AXIS2_PLACEMENT_3D ( 'NONE', #9325, #11542, #1239 ) ;
#2273=DIRECTION ( 'NONE',  ( -0.000000000000000000, -0.000000000000000000, -1.000000000000000000 ) ) ;
#2275=LINE ( 'NONE', #49, #1189 ) ;
#2283=VERTEX_POINT ( 'NONE', #1151 ) ;
#2285=EDGE_LOOP ( 'NONE', ( #11883, #9864, #9691, #10059 ) ) ;
#2287=ADVANCED_FACE ( 'NONE', ( #15012 ), #11382, .T. ) ;
#2294=ORIENTED_EDGE ( 'NONE', *, *, #1364, .F. ) ;
#2307=VERTEX_POINT ( 'NONE', #15093 ) ;
#2312=LINE ( 'NONE', #11690, #8406 ) ;
#2314=VERTEX_POINT ( 'NONE', #4542 ) ;
#2315=CARTESIAN_POINT ( 'NONE',  ( 118.0000000000000284, 23.25070940071369563, 33.00000000000012790 ) ) ;
#2326=CARTESIAN_POINT ( 'NONE',  ( 109.8334623555409735, 23.25070940071369563, 139.1143251403882459 ) ) ;
#2327=DIRECTION ( 'NONE',  ( 0.000000000000000000, 0.000000000000000000, 1.000000000000000000 ) ) ;
#2328=ORIENTED_EDGE ( 'NONE', *, *, #13643, .T. ) ;
#2335=DIRECTION ( 'NONE',  ( -1.000000000000000000, 0.000000000000000000, 0.000000000000000000 ) ) ;
#2350=CARTESIAN_POINT ( 'NONE',  ( -2.016677571526633510E-15, 23.25070940071368497, 33.00000000000012790 ) ) ;
#2352=ADVANCED_FACE ( 'NONE', ( #4623 ), #3158, .T. ) ;
#2356=ORIENTED_EDGE ( 'NONE', *, *, #6494, .T. ) ;
#2358=CARTESIAN_POINT ( 'NONE',  ( 118.0000000000000284, 23.25070940071369563, 13.14990448602692474 ) ) ;
#2365=LINE ( 'NONE', #138, #12596 ) ;
#2376=ORIENTED_EDGE ( 'NONE', *, *, #12041, .F. ) ;
#2392=AXIS2_PLACEMENT_3D ( 'NONE', #11950, #4573, #7115 ) ;
#2398=ORIENTED_EDGE ( 'NONE', *, *, #937, .F. ) ;
#2405=VECTOR ( 'NONE', #14297, 1000.000000000000000 ) ;
#2408=AXIS2_PLACEMENT_3D ( 'NONE', #6503, #11193, #642 ) ;
#2415=EDGE_CURVE ( 'NONE', #587, #13534, #7090, .T. ) ;
#2422=DIRECTION ( 'NONE',  ( -0.000000000000000000, -0.000000000000000000, -1.000000000000000000 ) ) ;
#2423=AXIS2_PLACEMENT_3D ( 'NONE', #10552, #13856, #9169 ) ;
#2424=ORIENTED_EDGE ( 'NONE', *, *, #1386, .F. ) ;
#2425=FACE_OUTER_BOUND ( 'NONE', #6698, .T. ) ;
#2426=CARTESIAN_POINT ( 'NONE',  ( 46.91810375148135392, 23.25070940071368852, 139.1143251403882459 ) ) ;
#2428=CARTESIAN_POINT ( 'NONE',  ( 88.00000000000001421, 10.75070940071369208, 139.1143251403882459 ) ) ;
#2433=EDGE_LOOP ( 'NONE', ( #13319, #2356, #3146, #4746 ) ) ;
#2436=DIRECTION ( 'NONE',  ( 0.000000000000000000, 1.000000000000000000, 0.000000000000000000 ) ) ;
#2448=VECTOR ( 'NONE', #4796, 1000.000000000000000 ) ;
#2452=LINE ( 'NONE', #6073, #12452 ) ;
#2460=EDGE_CURVE ( 'NONE', #20, #6460, #4929, .T. ) ;
#2464=VECTOR ( 'NONE', #1650, 1000.000000000000000 ) ;
#2469=LINE ( 'NONE', #10702, #4099 ) ;
#2472=ORIENTED_EDGE ( 'NONE', *, *, #647, .T. ) ;
#2474=VECTOR ( 'NONE', #6981, 1000.000000000000000 ) ;
#2476=CARTESIAN_POINT ( 'NONE',  ( 108.0866310645538562, 21.75070940071366365, -33.00000000000012790 ) ) ;
#2485=LINE ( 'NONE', #11874, #6953 ) ;
#2488=ORIENTED_EDGE ( 'NONE', *, *, #8437, .F. ) ;
#2492=PLANE ( 'NONE',  #7898 ) ;
#2497=CARTESIAN_POINT ( 'NONE',  ( -2.016677571526633510E-15, 23.25070940071368497, -33.00000000000012790 ) ) ;
#2498=DIRECTION ( 'NONE',  ( 1.000000000000000000, 0.000000000000000000, 0.000000000000000000 ) ) ;
#2501=EDGE_CURVE ( 'NONE', #14453, #2542, #1385, .T. ) ;
#2529=VECTOR ( 'NONE', #8977, 1000.000000000000000 ) ;
#2535=VERTEX_POINT ( 'NONE', #14396 ) ;
#2541=DIRECTION ( 'NONE',  ( -1.000000000000000000, 0.000000000000000000, 0.000000000000000000 ) ) ;
#2542=VERTEX_POINT ( 'NONE', #240 ) ;
#2544=CARTESIAN_POINT ( 'NONE',  ( 0.000000000000000000, 21.75070940071363168, -33.00000000000012790 ) ) ;
#2550=CARTESIAN_POINT ( 'NONE',  ( 0.000000000000000000, 21.75070940071312364, 33.00000000000012790 ) ) ;
#2551=DIRECTION ( 'NONE',  ( -0.000000000000000000, -0.000000000000000000, -1.000000000000000000 ) ) ;
#2556=ORIENTED_EDGE ( 'NONE', *, *, #6685, .T. ) ;
#2562=CARTESIAN_POINT ( 'NONE',  ( 42.07846078193830408, 0.000000000000000000, 33.00000000000012790 ) ) ;
#2563=VERTEX_POINT ( 'NONE', #7534 ) ;
#2590=CARTESIAN_POINT ( 'NONE',  ( -2.688903428702175252E-15, 23.25070940071368142, 139.1143251403882459 ) ) ;
#2597=VERTEX_POINT ( 'NONE', #12447 ) ;
#2598=ORIENTED_EDGE ( 'NONE', *, *, #222, .T. ) ;
#2600=CARTESIAN_POINT ( 'NONE',  ( -2.016677571526633510E-15, 23.25070940071368497, -33.00000000000012790 ) ) ;
#2602=ORIENTED_EDGE ( 'NONE', *, *, #6533, .T. ) ;
#2608=CARTESIAN_POINT ( 'NONE',  ( 51.75774672102440377, 21.75070940071325865, 33.00000000000012790 ) ) ;
#2611=DIRECTION ( 'NONE',  ( 1.000000000000000000, 0.000000000000000000, 0.000000000000000000 ) ) ;
#2613=ORIENTED_EDGE ( 'NONE', *, *, #7308, .F. ) ;
#2616=DIRECTION ( 'NONE',  ( 5.551115123125786646E-16, 1.000000000000000000, 0.000000000000000000 ) ) ;
#2620=LINE ( 'NONE', #2776, #4621 ) ;
#2625=EDGE_LOOP ( 'NONE', ( #838, #11779, #11928, #11061 ) ) ;
#2627=ORIENTED_EDGE ( 'NONE', *, *, #8772, .T. ) ;
#2629=CARTESIAN_POINT ( 'NONE',  ( 114.0000000000000284, 15.25070940071369563, -33.00000000000012790 ) ) ;
#2634=CARTESIAN_POINT ( 'NONE',  ( 0.000000000000000000, 21.75070940071366365, 139.1143251403882459 ) ) ;
#2635=CARTESIAN_POINT ( 'NONE',  ( 0.000000000000000000, 21.75070940071366365, 33.00000000000012790 ) ) ;
#2651=EDGE_CURVE ( 'NONE', #2283, #550, #4697, .T. ) ;
#2659=VECTOR ( 'NONE', #12566, 1000.000000000000000 ) ;
#2667=CARTESIAN_POINT ( 'NONE',  ( 88.00000000000000000, 23.25070940071369208, 139.1143251403882459 ) ) ;
#2668=CARTESIAN_POINT ( 'NONE',  ( 114.0000000000000284, 19.25070940071369563, 139.1143251403882459 ) ) ;
#2672=EDGE_CURVE ( 'NONE', #9539, #7261, #13379, .T. ) ;
#2680=ORIENTED_EDGE ( 'NONE', *, *, #1222, .T. ) ;
#2682=ORIENTED_EDGE ( 'NONE', *, *, #5724, .F. ) ;
#2685=ORIENTED_EDGE ( 'NONE', *, *, #5455, .T. ) ;
#2688=ORIENTED_EDGE ( 'NONE', *, *, #387, .T. ) ;
#2690=EDGE_CURVE ( 'NONE', #10867, #12323, #8965, .T. ) ;
#2702=VECTOR ( 'NONE', #7183, 1000.000000000000000 ) ;
#2705=CARTESIAN_POINT ( 'NONE',  ( 30.65234355186507997, 0.000000000000000000, 139.1143251403882459 ) ) ;
#2732=DIRECTION ( 'NONE',  ( 0.000000000000000000, 1.000000000000000000, -0.000000000000000000 ) ) ;
#2738=DIRECTION ( 'NONE',  ( -0.000000000000000000, -0.000000000000000000, -1.000000000000000000 ) ) ;
#2741=EDGE_CURVE ( 'NONE', #1838, #6910, #12749, .T. ) ;
#2745=EDGE_CURVE ( 'NONE', #10066, #14864, #10201, .T. ) ;
#2750=EDGE_CURVE ( 'NONE', #11132, #5929, #9048, .T. ) ;
#2757=ORIENTED_EDGE ( 'NONE', *, *, #8397, .F. ) ;
#2766=VECTOR ( 'NONE', #14999, 1000.000000000000000 ) ;
#2776=CARTESIAN_POINT ( 'NONE',  ( 45.17127246049422240, 23.25070940071368852, 139.1143251403882459 ) ) ;
#2778=ORIENTED_EDGE ( 'NONE', *, *, #7068, .F. ) ;
#2794=LINE ( 'NONE', #12329, #9851 ) ;
#2796=ORIENTED_EDGE ( 'NONE', *, *, #3559, .F. ) ;
#2801=DIRECTION ( 'NONE',  ( -0.000000000000000000, -0.000000000000000000, -1.000000000000000000 ) ) ;
#2812=LINE ( 'NONE', #14439, #54 ) ;
#2813=ORIENTED_EDGE ( 'NONE', *, *, #12339, .T. ) ;
#2815=DIRECTION ( 'NONE',  ( -1.000000000000000000, -8.673617379884035472E-17, 0.000000000000000000 ) ) ;
#2816=CARTESIAN_POINT ( 'NONE',  ( 112.9262740340969060, 0.000000000000000000, -13.14990448602693007 ) ) ;
#2820=EDGE_CURVE ( 'NONE', #6214, #8236, #15052, .T. ) ;
#2821=ORIENTED_EDGE ( 'NONE', *, *, #4449, .F. ) ;
#2839=VECTOR ( 'NONE', #1697, 1000.000000000000000 ) ;
#2840=CARTESIAN_POINT ( 'NONE',  ( 114.6731053250840233, 21.75070940071369918, 33.00000000000012790 ) ) ;
#2841=ORIENTED_EDGE ( 'NONE', *, *, #7619, .F. ) ;
#2843=DIRECTION ( 'NONE',  ( 0.000000000000000000, 1.000000000000000000, -0.000000000000000000 ) ) ;
#2847=VECTOR ( 'NONE', #17, 1000.000000000000000 ) ;
#2852=CARTESIAN_POINT ( 'NONE',  ( 104.0000000000000426, 11.25070940071369563, -33.00000000000014211 ) ) ;
#2853=DIRECTION ( 'NONE',  ( -0.000000000000000000, -0.000000000000000000, -1.000000000000000000 ) ) ;
#2856=DIRECTION ( 'NONE',  ( -1.000000000000000000, 0.000000000000000000, 0.000000000000000000 ) ) ;
#2869=DIRECTION ( 'NONE',  ( 1.000000000000000000, 8.673617379884035472E-17, 0.000000000000000000 ) ) ;
#2872=CARTESIAN_POINT ( 'NONE',  ( 103.2469880950108063, 21.75070940071363168, -33.00000000000012790 ) ) ;
#2873=ORIENTED_EDGE ( 'NONE', *, *, #9606, .T. ) ;
#2881=LINE ( 'NONE', #13499, #6694 ) ;
#2883=EDGE_LOOP ( 'NONE', ( #10438, #4917, #8801, #2841 ) ) ;
#2899=CARTESIAN_POINT ( 'NONE',  ( 114.6731053250840233, 0.000000000000000000, 139.1143251403882459 ) ) ;
#2900=VECTOR ( 'NONE', #12536, 1000.000000000000000 ) ;
#2904=ORIENTED_EDGE ( 'NONE', *, *, #2745, .F. ) ;
#2906=CARTESIAN_POINT ( 'NONE',  ( 0.000000000000000000, 21.75070940071315562, 33.00000000000012790 ) ) ;
#2916=CARTESIAN_POINT ( 'NONE',  ( -2.016677571526633510E-15, 23.25070940071368497, 139.1143251403882459 ) ) ;
#2918=CARTESIAN_POINT ( 'NONE',  ( 50.01091543003727224, 21.75070940071325865, -33.00000000000012790 ) ) ;
#2921=ORIENTED_EDGE ( 'NONE', *, *, #11765, .F. ) ;
#2926=FACE_OUTER_BOUND ( 'NONE', #7899, .T. ) ;
#2932=ORIENTED_EDGE ( 'NONE', *, *, #2144, .T. ) ;
#2933=LINE ( 'NONE', #7625, #11739 ) ;
#2950=ORIENTED_EDGE ( 'NONE', *, *, #11121, .F. ) ;
#2955=( NAMED_UNIT ( * ) SI_UNIT ( $, .STERADIAN. ) SOLID_ANGLE_UNIT ( ) );
#2960=ORIENTED_EDGE ( 'NONE', *, *, #1567, .F. ) ;
#2967=EDGE_CURVE ( 'NONE', #1905, #14376, #12036, .T. ) ;
#2969=ORIENTED_EDGE ( 'NONE', *, *, #4653, .F. ) ;
#2973=CARTESIAN_POINT ( 'NONE',  ( 105.5545870572953930, 23.25070940071369563, 13.14990448602692474 ) ) ;
#2975=VERTEX_POINT ( 'NONE', #12182 ) ;
#2986=CARTESIAN_POINT ( 'NONE',  ( 51.75774672102440377, 23.25070940071368852, 139.1143251403882459 ) ) ;
#2993=VECTOR ( 'NONE', #11770, 1000.000000000000000 ) ;
#3001=EDGE_LOOP ( 'NONE', ( #13316, #731, #1779, #1003 ) ) ;
#3009=CARTESIAN_POINT ( 'NONE',  ( -2.688903428702175252E-15, 23.25070940071368142, 139.1143251403882459 ) ) ;
#3013=AXIS2_PLACEMENT_3D ( 'NONE', #2590, #12991, #11671 ) ;
#3014=DIRECTION ( 'NONE',  ( -1.000000000000000000, -1.734723475976807292E-15, 0.000000000000000000 ) ) ;
#3015=CARTESIAN_POINT ( 'NONE',  ( 40.33162949095117966, 21.75070940071319114, 33.00000000000012790 ) ) ;
#3017=VECTOR ( 'NONE', #6861, 1000.000000000000000 ) ;
#3039=VECTOR ( 'NONE', #6310, 1000.000000000000000 ) ;
#3043=ORIENTED_EDGE ( 'NONE', *, *, #11823, .F. ) ;
#3048=CARTESIAN_POINT ( 'NONE',  ( 108.0866310645538562, 21.75070940071366365, -13.14990448602693007 ) ) ;
#3064=ORIENTED_EDGE ( 'NONE', *, *, #10647, .F. ) ;
#3077=CARTESIAN_POINT ( 'NONE',  ( 0.000000000000000000, 21.75070940071366365, -33.00000000000012790 ) ) ;
#3078=CARTESIAN_POINT ( 'NONE',  ( 35.49198652140812982, 0.000000000000000000, -33.00000000000012790 ) ) ;
#3079=ORIENTED_EDGE ( 'NONE', *, *, #6532, .T. ) ;
#3085=ORIENTED_EDGE ( 'NONE', *, *, #5702, .T. ) ;
#3088=EDGE_LOOP ( 'NONE', ( #15197, #7111, #13663, #4211 ) ) ;
#3093=ORIENTED_EDGE ( 'NONE', *, *, #12852, .F. ) ;
#3101=ORIENTED_EDGE ( 'NONE', *, *, #8041, .F. ) ;
#3102=EDGE_CURVE ( 'NONE', #13132, #4131, #10107, .T. ) ;
#3104=LINE ( 'NONE', #4329, #14070 ) ;
#3123=LINE ( 'NONE', #12142, #1401 ) ;
#3126=EDGE_LOOP ( 'NONE', ( #3043, #2097, #8837, #5912 ) ) ;
#3131=CARTESIAN_POINT ( 'NONE',  ( 37.23881781239525424, 0.000000000000000000, 33.00000000000012790 ) ) ;
#3138=CYLINDRICAL_SURFACE ( 'NONE', #13502, 4.000000000000003553 ) ;
#3145=PLANE ( 'NONE',  #12481 ) ;
#3146=ORIENTED_EDGE ( 'NONE', *, *, #6594, .F. ) ;
#3150=ORIENTED_EDGE ( 'NONE', *, *, #13449, .T. ) ;
#3155=LINE ( 'NONE', #11300, #5068 ) ;
#3158=PLANE ( 'NONE',  #8151 ) ;
#3163=DIRECTION ( 'NONE',  ( 0.000000000000000000, 0.000000000000000000, 1.000000000000000000 ) ) ;
#3164=FACE_OUTER_BOUND ( 'NONE', #7169, .T. ) ;
#3167=CARTESIAN_POINT ( 'NONE',  ( 43.00000000000000711, 10.25070940071368497, 33.00000000000012790 ) ) ;
#3178=PLANE ( 'NONE',  #12328 ) ;
#3184=ORIENTED_EDGE ( 'NONE', *, *, #7284, .F. ) ;
#3192=CARTESIAN_POINT ( 'NONE',  ( 118.0000000000000568, 2.046973701652633381E-13, -33.00000000000012790 ) ) ;
#3194=EDGE_CURVE ( 'NONE', #5487, #2975, #110, .T. ) ;
#3195=LINE ( 'NONE', #2973, #12889 ) ;
#3196=LINE ( 'NONE', #7895, #9280 ) ;
#3205=DIRECTION ( 'NONE',  ( -0.000000000000000000, -0.000000000000000000, -1.000000000000000000 ) ) ;
#3210=EDGE_CURVE ( 'NONE', #7396, #1788, #8190, .T. ) ;
#3221=ORIENTED_EDGE ( 'NONE', *, *, #12327, .F. ) ;
#3224=AXIS2_PLACEMENT_3D ( 'NONE', #10041, #1866, #11406 ) ;
#3225=FACE_OUTER_BOUND ( 'NONE', #5552, .T. ) ;
#3229=LINE ( 'NONE', #914, #11845 ) ;
#3245=DIRECTION ( 'NONE',  ( 1.000000000000000000, 0.000000000000000000, 0.000000000000000000 ) ) ;
#3250=CARTESIAN_POINT ( 'NONE',  ( -2.016677571526633510E-15, 23.25070940071368497, 139.1143251403882459 ) ) ;
#3253=VECTOR ( 'NONE', #4554, 1000.000000000000000 ) ;
#3259=ADVANCED_FACE ( 'NONE', ( #12958 ), #11871, .T. ) ;
#3266=LINE ( 'NONE', #10114, #10605 ) ;
#3269=VERTEX_POINT ( 'NONE', #2252 ) ;
#3275=DIRECTION ( 'NONE',  ( -1.734723475976807094E-15, 1.000000000000000000, 0.000000000000000000 ) ) ;
#3278=CARTESIAN_POINT ( 'NONE',  ( 0.000000000000000000, 15.25070940071368497, 33.00000000000012790 ) ) ;
#3283=CARTESIAN_POINT ( 'NONE',  ( 62.00000000000001421, -2.249290599286310588, -33.00000000000012790 ) ) ;
#3286=DIRECTION ( 'NONE',  ( -0.000000000000000000, -0.000000000000000000, -1.000000000000000000 ) ) ;
#3297=ORIENTED_EDGE ( 'NONE', *, *, #7639, .F. ) ;
#3303=EDGE_CURVE ( 'NONE', #7451, #4834, #6377, .T. ) ;
#3305=PLANE ( 'NONE',  #12861 ) ;
#3308=CYLINDRICAL_SURFACE ( 'NONE', #11587, 4.000000000000003553 ) ;
#3323=CARTESIAN_POINT ( 'NONE',  ( 40.33162949095117966, 0.000000000000000000, 33.00000000000012790 ) ) ;
#3326=LINE ( 'NONE', #778, #4567 ) ;
#3328=EDGE_CURVE ( 'NONE', #1460, #4646, #12250, .T. ) ;
#3341=FACE_OUTER_BOUND ( 'NONE', #2167, .T. ) ;
#3344=EDGE_CURVE ( 'NONE', #4786, #72, #8560, .T. ) ;
#3349=DIRECTION ( 'NONE',  ( -0.000000000000000000, -0.000000000000000000, -1.000000000000000000 ) ) ;
#3364=ORIENTED_EDGE ( 'NONE', *, *, #14266, .T. ) ;
#3373=ORIENTED_EDGE ( 'NONE', *, *, #5898, .F. ) ;
#3377=ORIENTED_EDGE ( 'NONE', *, *, #5054, .F. ) ;
#3383=FACE_OUTER_BOUND ( 'NONE', #11906, .T. ) ;
#3390=ADVANCED_FACE ( 'NONE', ( #11164 ), #5168, .F. ) ;
#3398=CARTESIAN_POINT ( 'NONE',  ( 0.000000000000000000, 21.75070940071325865, -33.00000000000012790 ) ) ;
#3399=EDGE_CURVE ( 'NONE', #5759, #10066, #9805, .T. ) ;
#3404=VERTEX_POINT ( 'NONE', #3932 ) ;
#3406=VECTOR ( 'NONE', #1920, 1000.000000000000000 ) ;
#3410=CARTESIAN_POINT ( 'NONE',  ( 93.56770215592470663, 21.75070940071356418, 33.00000000000012790 ) ) ;
#3415=ORIENTED_EDGE ( 'NONE', *, *, #12379, .T. ) ;
#3429=DIRECTION ( 'NONE',  ( -1.000000000000000000, -8.673617379884035472E-17, 0.000000000000000000 ) ) ;
#3431=LINE ( 'NONE', #1037, #13598 ) ;
#3434=LINE ( 'NONE', #8289, #6808 ) ;
#3441=DIRECTION ( 'NONE',  ( 0.000000000000000000, 1.000000000000000000, -0.000000000000000000 ) ) ;
#3442=ORIENTED_EDGE ( 'NONE', *, *, #14415, .T. ) ;
#3443=CARTESIAN_POINT ( 'NONE',  ( 58.00000000000000711, -2.249290599286307479, 139.1143251403882459 ) ) ;
#3444=CARTESIAN_POINT ( 'NONE',  ( 58.00000000000000711, -2.249290599286307479, -33.00000000000012790 ) ) ;
#3453=EDGE_CURVE ( 'NONE', #5614, #6214, #9170, .T. ) ;
#3456=EDGE_LOOP ( 'NONE', ( #265, #2688 ) ) ;
#3458=ORIENTED_EDGE ( 'NONE', *, *, #14907, .F. ) ;
#3459=ORIENTED_EDGE ( 'NONE', *, *, #5702, .F. ) ;
#3461=DIRECTION ( 'NONE',  ( -1.000000000000000000, -1.156482317317870492E-16, 0.000000000000000000 ) ) ;
#3466=ORIENTED_EDGE ( 'NONE', *, *, #449, .T. ) ;
#3471=DIRECTION ( 'NONE',  ( 5.551115123125787632E-16, 1.000000000000000000, -0.000000000000000000 ) ) ;
#3473=LINE ( 'NONE', #10556, #3881 ) ;
#3476=DIRECTION ( 'NONE',  ( 0.000000000000000000, 1.000000000000000000, 0.000000000000000000 ) ) ;
#3477=CARTESIAN_POINT ( 'NONE',  ( 0.000000000000000000, 21.75070940071366365, -13.14990448602693007 ) ) ;
#3483=CYLINDRICAL_SURFACE ( 'NONE', #5303, 4.999999999999997335 ) ;
#3485=ADVANCED_FACE ( 'NONE', ( #13857 ), #7860, .F. ) ;
#3486=VECTOR ( 'NONE', #3808, 1000.000000000000000 ) ;
#3504=VECTOR ( 'NONE', #2422, 1000.000000000000000 ) ;
#3507=ADVANCED_FACE ( 'NONE', ( #7257 ), #4876, .F. ) ;
#3510=DIRECTION ( 'NONE',  ( 1.000000000000000000, 0.000000000000000000, 0.000000000000000000 ) ) ;
#3513=VECTOR ( 'NONE', #359, 1000.000000000000000 ) ;
#3519=ORIENTED_EDGE ( 'NONE', *, *, #4576, .F. ) ;
#3523=PLANE ( 'NONE',  #3013 ) ;
#3529=VECTOR ( 'NONE', #2551, 1000.000000000000000 ) ;
#3533=EDGE_LOOP ( 'NONE', ( #13004, #3810, #10052, #7458 ) ) ;
#3539=VECTOR ( 'NONE', #11207, 1000.000000000000000 ) ;
#3541=DIRECTION ( 'NONE',  ( 0.000000000000000000, -0.000000000000000000, 1.000000000000000000 ) ) ;
#3549=DIRECTION ( 'NONE',  ( -0.000000000000000000, -0.000000000000000000, -1.000000000000000000 ) ) ;
#3553=FACE_OUTER_BOUND ( 'NONE', #2625, .T. ) ;
#3558=ORIENTED_EDGE ( 'NONE', *, *, #4630, .T. ) ;
#3559=EDGE_CURVE ( 'NONE', #14644, #7451, #9875, .T. ) ;
#3565=CARTESIAN_POINT ( 'NONE',  ( 109.8334623555409735, 21.75070940071366365, 139.1143251403882459 ) ) ;
#3568=EDGE_CURVE ( 'NONE', #322, #11132, #8854, .T. ) ;
#3571=FACE_OUTER_BOUND ( 'NONE', #6982, .T. ) ;
#3572=CARTESIAN_POINT ( 'NONE',  ( 112.9262740340969060, 23.25070940071369563, -33.00000000000012790 ) ) ;
#3582=EDGE_LOOP ( 'NONE', ( #10686, #10805, #14708, #8367 ) ) ;
#3608=EDGE_CURVE ( 'NONE', #5719, #5383, #4462, .T. ) ;
#3614=CARTESIAN_POINT ( 'NONE',  ( 100.0000000000000284, 6.750709400713692965, -33.00000000000012790 ) ) ;
#3621=CIRCLE ( 'NONE', #3853, 4.000000000000003553 ) ;
#3630=EDGE_CURVE ( 'NONE', #12374, #13354, #13273, .T. ) ;
#3647=VECTOR ( 'NONE', #4704, 1000.000000000000000 ) ;
#3648=ORIENTED_EDGE ( 'NONE', *, *, #1567, .T. ) ;
#3654=PLANE ( 'NONE',  #6204 ) ;
#3657=DIRECTION ( 'NONE',  ( 0.000000000000000000, 1.000000000000000000, -0.000000000000000000 ) ) ;
#3661=CARTESIAN_POINT ( 'NONE',  ( 25.81270058232203013, 0.000000000000000000, 33.00000000000012790 ) ) ;
#3665=DIRECTION ( 'NONE',  ( 1.000000000000000000, 0.000000000000000000, 0.000000000000000000 ) ) ;
#3666=VERTEX_POINT ( 'NONE', #5685 ) ;
#3685=ORIENTED_EDGE ( 'NONE', *, *, #6598, .F. ) ;
#3689=EDGE_CURVE ( 'NONE', #550, #13470, #14991, .T. ) ;
#3693=ORIENTED_EDGE ( 'NONE', *, *, #1457, .F. ) ;
#3694=DIRECTION ( 'NONE',  ( -0.000000000000000000, -0.000000000000000000, -1.000000000000000000 ) ) ;
#3700=ORIENTED_EDGE ( 'NONE', *, *, #3194, .T. ) ;
#3703=ORIENTED_EDGE ( 'NONE', *, *, #14732, .F. ) ;
#3708=DIRECTION ( 'NONE',  ( 0.000000000000000000, 0.000000000000000000, 1.000000000000000000 ) ) ;
#3709=DIRECTION ( 'NONE',  ( -0.000000000000000000, -0.000000000000000000, -1.000000000000000000 ) ) ;
#3721=CARTESIAN_POINT ( 'NONE',  ( 100.1541764164548880, 0.000000000000000000, 33.00000000000012790 ) ) ;
#3733=LINE ( 'NONE', #6134, #12784 ) ;
#3742=CARTESIAN_POINT ( 'NONE',  ( 46.91810375148135392, 0.000000000000000000, -33.00000000000012790 ) ) ;
#3746=AXIS2_PLACEMENT_3D ( 'NONE', #2899, #588, #5289 ) ;
#3753=DIRECTION ( 'NONE',  ( 1.000000000000000000, 0.000000000000000000, 0.000000000000000000 ) ) ;
#3758=CIRCLE ( 'NONE', #12356, 4.000000000000003553 ) ;
#3761=CARTESIAN_POINT ( 'NONE',  ( 37.23881781239525424, 21.75070940071315562, 33.00000000000012790 ) ) ;
#3768=ORIENTED_EDGE ( 'NONE', *, *, #4630, .F. ) ;
#3776=ADVANCED_FACE ( 'NONE', ( #8981 ), #3138, .F. ) ;
#3779=LINE ( 'NONE', #4859, #11594 ) ;
#3808=DIRECTION ( 'NONE',  ( 1.000000000000000000, 0.000000000000000000, 0.000000000000000000 ) ) ;
#3810=ORIENTED_EDGE ( 'NONE', *, *, #9661, .T. ) ;
#3813=EDGE_CURVE ( 'NONE', #9928, #3922, #8645, .T. ) ;
#3819=CARTESIAN_POINT ( 'NONE',  ( 100.1541764164548880, 0.000000000000000000, 139.1143251403882459 ) ) ;
#3824=ORIENTED_EDGE ( 'NONE', *, *, #5099, .T. ) ;
#3832=LINE ( 'NONE', #2906, #1632 ) ;
#3840=ORIENTED_EDGE ( 'NONE', *, *, #6598, .T. ) ;
#3842=ORIENTED_EDGE ( 'NONE', *, *, #2690, .F. ) ;
#3849=ADVANCED_FACE ( 'NONE', ( #5844 ), #352, .F. ) ;
#3853=AXIS2_PLACEMENT_3D ( 'NONE', #14819, #6364, #11129 ) ;
#3873=EDGE_CURVE ( 'NONE', #5614, #8184, #14871, .T. ) ;
#3874=AXIS2_PLACEMENT_3D ( 'NONE', #2705, #7699, #8844 ) ;
#3877=ADVANCED_FACE ( 'NONE', ( #13723 ), #3178, .F. ) ;
#3881=VECTOR ( 'NONE', #6935, 1000.000000000000000 ) ;
#3882=VECTOR ( 'NONE', #14886, 1000.000000000000000 ) ;
#3884=FACE_OUTER_BOUND ( 'NONE', #4685, .T. ) ;
#3885=EDGE_LOOP ( 'NONE', ( #3768, #12110, #1367, #5122 ) ) ;
#3890=ORIENTED_EDGE ( 'NONE', *, *, #14215, .T. ) ;
#3893=EDGE_LOOP ( 'NONE', ( #130, #380, #11295, #4351 ) ) ;
#3906=ORIENTED_EDGE ( 'NONE', *, *, #11823, .T. ) ;
#3909=ORIENTED_EDGE ( 'NONE', *, *, #13049, .T. ) ;
#3911=ORIENTED_EDGE ( 'NONE', *, *, #9809, .T. ) ;
#3912=VECTOR ( 'NONE', #14485, 1000.000000000000000 ) ;
#3922=VERTEX_POINT ( 'NONE', #13878 ) ;
#3925=VERTEX_POINT ( 'NONE', #8270 ) ;
#3932=CARTESIAN_POINT ( 'NONE',  ( 54.85055839958032209, 23.25070940071368852, -33.00000000000012790 ) ) ;
#3948=VECTOR ( 'NONE', #13738, 1000.000000000000000 ) ;
#3952=EDGE_CURVE ( 'NONE', #10066, #2563, #14113, .T. ) ;
#3968=VERTEX_POINT ( 'NONE', #8110 ) ;
#3987=CARTESIAN_POINT ( 'NONE',  ( 105.5545870572953930, -1.749290599286305259, 13.14990448602692474 ) ) ;
#3999=LINE ( 'NONE', #14693, #66 ) ;
#4014=ADVANCED_FACE ( 'NONE', ( #32 ), #6717, .T. ) ;
#4016=AXIS2_PLACEMENT_3D ( 'NONE', #14085, #8242, #7082 ) ;
#4030=CARTESIAN_POINT ( 'NONE',  ( 48.00000000000000000, -2.249290599286307479, 33.00000000000012790 ) ) ;
#4047=FACE_OUTER_BOUND ( 'NONE', #5621, .T. ) ;
#4054=DIRECTION ( 'NONE',  ( 1.000000000000000000, 0.000000000000000000, 0.000000000000000000 ) ) ;
#4057=ORIENTED_EDGE ( 'NONE', *, *, #8623, .T. ) ;
#4060=EDGE_CURVE ( 'NONE', #10618, #1834, #9970, .T. ) ;
#4061=ORIENTED_EDGE ( 'NONE', *, *, #9606, .F. ) ;
#4063=CARTESIAN_POINT ( 'NONE',  ( 104.0000000000000426, 15.25070940071369563, 33.00000000000012790 ) ) ;
#4069=PLANE ( 'NONE',  #13471 ) ;
#4071=DIRECTION ( 'NONE',  ( -0.000000000000000000, 0.000000000000000000, 1.000000000000000000 ) ) ;
#4074=DIRECTION ( 'NONE',  ( -1.000000000000000000, 0.000000000000000000, 0.000000000000000000 ) ) ;
#4077=AXIS2_PLACEMENT_3D ( 'NONE', #9848, #13373, #9987 ) ;
#4082=CARTESIAN_POINT ( 'NONE',  ( 0.000000000000000000, 0.000000000000000000, 0.000000000000000000 ) ) ;
#4084=VERTEX_POINT ( 'NONE', #9122 ) ;
#4085=VECTOR ( 'NONE', #3753, 1000.000000000000000 ) ;
#4087=VECTOR ( 'NONE', #9353, 1000.000000000000000 ) ;
#4099=VECTOR ( 'NONE', #8005, 1000.000000000000000 ) ;
#4100=ORIENTED_EDGE ( 'NONE', *, *, #7567, .T. ) ;
#4119=EDGE_CURVE ( 'NONE', #4131, #14644, #7901, .T. ) ;
#4122=AXIS2_PLACEMENT_3D ( 'NONE', #12400, #4074, #3163 ) ;
#4126=VECTOR ( 'NONE', #11890, 1000.000000000000000 ) ;
#4131=VERTEX_POINT ( 'NONE', #4500 ) ;
#4147=VECTOR ( 'NONE', #10490, 1000.000000000000000 ) ;
#4154=DIRECTION ( 'NONE',  ( 1.000000000000000000, 0.000000000000000000, 0.000000000000000000 ) ) ;
#4161=ORIENTED_EDGE ( 'NONE', *, *, #10247, .F. ) ;
#4171=CARTESIAN_POINT ( 'NONE',  ( 68.00000000000001421, 1.887379141862766624E-13, 139.1143251403882459 ) ) ;
#4187=LINE ( 'NONE', #7743, #7075 ) ;
#4191=ORIENTED_EDGE ( 'NONE', *, *, #5015, .F. ) ;
#4206=AXIS2_PLACEMENT_3D ( 'NONE', #6205, #12116, #5181 ) ;
#4210=CARTESIAN_POINT ( 'NONE',  ( 25.81270058232203013, 0.000000000000000000, -33.00000000000012790 ) ) ;
#4211=ORIENTED_EDGE ( 'NONE', *, *, #8572, .F. ) ;
#4231=AXIS2_PLACEMENT_3D ( 'NONE', #3009, #6531, #6611 ) ;
#4235=AXIS2_PLACEMENT_3D ( 'NONE', #3444, #10978, #13215 ) ;
#4237=VERTEX_POINT ( 'NONE', #7343 ) ;
#4259=CARTESIAN_POINT ( 'NONE',  ( -2.016677571526633510E-15, 23.25070940071368497, 33.00000000000012790 ) ) ;
#4269=ADVANCED_FACE ( 'NONE', ( #411 ), #6125, .F. ) ;
#4274=LINE ( 'NONE', #10061, #13669 ) ;
#4279=ORIENTED_EDGE ( 'NONE', *, *, #6928, .F. ) ;
#4283=DIRECTION ( 'NONE',  ( 8.673617379884035472E-17, -1.000000000000000000, 0.000000000000000000 ) ) ;
#4284=ORIENTED_EDGE ( 'NONE', *, *, #8437, .T. ) ;
#4285=VERTEX_POINT ( 'NONE', #10892 ) ;
#4290=LINE ( 'NONE', #980, #7928 ) ;
#4292=ORIENTED_EDGE ( 'NONE', *, *, #14114, .T. ) ;
#4310=FACE_OUTER_BOUND ( 'NONE', #3893, .T. ) ;
#4320=CARTESIAN_POINT ( 'NONE',  ( 40.33162949095117966, 23.25070940071368852, 33.00000000000012790 ) ) ;
#4326=CARTESIAN_POINT ( 'NONE',  ( 42.07846078193830408, 23.25070940071368852, 33.00000000000012790 ) ) ;
#4329=CARTESIAN_POINT ( 'NONE',  ( 130.4454129427046496, 23.25070940071369563, 13.14990448602692474 ) ) ;
#4331=LINE ( 'NONE', #2031, #15067 ) ;
#4335=ADVANCED_FACE ( 'NONE', ( #836 ), #3308, .T. ) ;
#4336=VECTOR ( 'NONE', #9451, 1000.000000000000000 ) ;
#4338=CARTESIAN_POINT ( 'NONE',  ( 88.00000000000000000, 23.25070940071369208, 33.00000000000012790 ) ) ;
#4339=CARTESIAN_POINT ( 'NONE',  ( 43.00000000000000711, 15.25070940071368497, -33.00000000000012790 ) ) ;
#4345=LINE ( 'NONE', #12593, #5853 ) ;
#4346=VERTEX_POINT ( 'NONE', #8002 ) ;
#4351=ORIENTED_EDGE ( 'NONE', *, *, #14436, .T. ) ;
#4363=ORIENTED_EDGE ( 'NONE', *, *, #12415, .F. ) ;
#4375=PRODUCT_DEFINITION_SHAPE ( 'NONE', 'NONE',  #9858 ) ;
#4376=AXIS2_PLACEMENT_3D ( 'NONE', #10736, #8283, #3510 ) ;
#4385=EDGE_CURVE ( 'NONE', #2563, #6792, #3229, .T. ) ;
#4396=VERTEX_POINT ( 'NONE', #2149 ) ;
#4397=CARTESIAN_POINT ( 'NONE',  ( -2.016677571526633510E-15, 23.25070940071368497, -33.00000000000012790 ) ) ;
#4399=ORIENTED_EDGE ( 'NONE', *, *, #7253, .T. ) ;
#4411=LINE ( 'NONE', #9035, #13563 ) ;
#4414=CARTESIAN_POINT ( 'NONE',  ( 48.00000000000000711, 10.25070940071368497, 139.1143251403882459 ) ) ;
#4415=EDGE_CURVE ( 'NONE', #7393, #4644, #6925, .T. ) ;
#4429=LINE ( 'NONE', #14821, #13782 ) ;
#4446=ORIENTED_EDGE ( 'NONE', *, *, #11196, .F. ) ;
#4449=EDGE_CURVE ( 'NONE', #13684, #9198, #8083, .T. ) ;
#4453=ORIENTED_EDGE ( 'NONE', *, *, #3399, .F. ) ;
#4457=DIRECTION ( 'NONE',  ( -1.000000000000000000, 0.000000000000000000, 0.000000000000000000 ) ) ;
#4460=DIRECTION ( 'NONE',  ( 0.000000000000000000, 1.000000000000000000, -0.000000000000000000 ) ) ;
#4462=LINE ( 'NONE', #2236, #11283 ) ;
#4467=VECTOR ( 'NONE', #10235, 1000.000000000000000 ) ;
#4474=ORIENTED_EDGE ( 'NONE', *, *, #12230, .F. ) ;
#4476=CARTESIAN_POINT ( 'NONE',  ( 112.9262740340969060, 21.75070940071369918, -33.00000000000012790 ) ) ;
#4500=CARTESIAN_POINT ( 'NONE',  ( 100.0000000000000284, 11.25070940071369563, 33.00000000000012790 ) ) ;
#4511=CARTESIAN_POINT ( 'NONE',  ( 42.07846078193830408, 21.75070940071319114, -33.00000000000012790 ) ) ;
#4517=CARTESIAN_POINT ( 'NONE',  ( 0.000000000000000000, 2.750709400713692965, -33.00000000000012790 ) ) ;
#4520=ADVANCED_FACE ( 'NONE', ( #8326 ), #11847, .F. ) ;
#4526=CARTESIAN_POINT ( 'NONE',  ( 35.49198652140812982, 21.75070940071315562, 33.00000000000012790 ) ) ;
#4533=ORIENTED_EDGE ( 'NONE', *, *, #2745, .T. ) ;
#4536=DIRECTION ( 'NONE',  ( 1.000000000000000000, 0.000000000000000000, 0.000000000000000000 ) ) ;
#4542=CARTESIAN_POINT ( 'NONE',  ( 114.6731053250840233, 21.75070940071369918, -33.00000000000012790 ) ) ;
#4553=LINE ( 'NONE', #4397, #7080 ) ;
#4554=DIRECTION ( 'NONE',  ( 1.000000000000000000, 0.000000000000000000, 0.000000000000000000 ) ) ;
#4557=DIRECTION ( 'NONE',  ( 1.000000000000000000, 8.673617379884035472E-17, 0.000000000000000000 ) ) ;
#4567=VECTOR ( 'NONE', #10183, 1000.000000000000000 ) ;
#4570=CARTESIAN_POINT ( 'NONE',  ( 104.9938193859979236, 0.000000000000000000, 139.1143251403882459 ) ) ;
#4573=DIRECTION ( 'NONE',  ( -1.000000000000000000, 0.000000000000000000, 0.000000000000000000 ) ) ;
#4576=EDGE_CURVE ( 'NONE', #12374, #13613, #10776, .T. ) ;
#4585=ORIENTED_EDGE ( 'NONE', *, *, #8487, .T. ) ;
#4593=VECTOR ( 'NONE', #8235, 1000.000000000000000 ) ;
#4602=LINE ( 'NONE', #12533, #9696 ) ;
#4604=ORIENTED_EDGE ( 'NONE', *, *, #1813, .T. ) ;
#4609=ORIENTED_EDGE ( 'NONE', *, *, #12041, .T. ) ;
#4610=VECTOR ( 'NONE', #1150, 1000.000000000000000 ) ;
#4615=PLANE ( 'NONE',  #1288 ) ;
#4620=VERTEX_POINT ( 'NONE', #14863 ) ;
#4621=VECTOR ( 'NONE', #461, 1000.000000000000000 ) ;
#4623=FACE_OUTER_BOUND ( 'NONE', #1524, .T. ) ;
#4630=EDGE_CURVE ( 'NONE', #6102, #8969, #15105, .T. ) ;
#4632=FACE_OUTER_BOUND ( 'NONE', #8135, .T. ) ;
#4638=LINE ( 'NONE', #9019, #8728 ) ;
#4639=CARTESIAN_POINT ( 'NONE',  ( 108.0866310645538562, 0.000000000000000000, 139.1143251403882459 ) ) ;
#4644=VERTEX_POINT ( 'NONE', #4476 ) ;
#4646=VERTEX_POINT ( 'NONE', #8021 ) ;
#4648=DIRECTION ( 'NONE',  ( 0.000000000000000000, 0.000000000000000000, 1.000000000000000000 ) ) ;
#4651=DIRECTION ( 'NONE',  ( 1.000000000000000000, 0.000000000000000000, 0.000000000000000000 ) ) ;
#4653=EDGE_CURVE ( 'NONE', #9290, #9928, #14788, .T. ) ;
#4655=EDGE_CURVE ( 'NONE', #8078, #7393, #5407, .T. ) ;
#4667=CARTESIAN_POINT ( 'NONE',  ( 58.00000000000000711, -2.249290599286311032, -33.00000000000012790 ) ) ;
#4677=VECTOR ( 'NONE', #11390, 1000.000000000000000 ) ;
#4681=LINE ( 'NONE', #13682, #6092 ) ;
#4683=ORIENTED_EDGE ( 'NONE', *, *, #12171, .F. ) ;
#4685=EDGE_LOOP ( 'NONE', ( #8803, #6903, #3415, #10373 ) ) ;
#4687=ORIENTED_EDGE ( 'NONE', *, *, #2672, .T. ) ;
#4690=DIRECTION ( 'NONE',  ( 1.000000000000000000, 0.000000000000000000, 0.000000000000000000 ) ) ;
#4697=CIRCLE ( 'NONE', #1501, 4.000000000000003553 ) ;
#4703=ORIENTED_EDGE ( 'NONE', *, *, #1705, .T. ) ;
#4704=DIRECTION ( 'NONE',  ( -0.000000000000000000, -0.000000000000000000, -1.000000000000000000 ) ) ;
#4712=CARTESIAN_POINT ( 'NONE',  ( 98.40734512546775647, 23.25070940071369208, 33.00000000000012790 ) ) ;
#4713=ORIENTED_EDGE ( 'NONE', *, *, #10946, .T. ) ;
#4716=EDGE_CURVE ( 'NONE', #11141, #8798, #6782, .T. ) ;
#4721=VECTOR ( 'NONE', #8325, 1000.000000000000000 ) ;
#4729=VERTEX_POINT ( 'NONE', #6944 ) ;
#4736=AXIS2_PLACEMENT_3D ( 'NONE', #930, #10331, #2327 ) ;
#4746=ORIENTED_EDGE ( 'NONE', *, *, #13449, .F. ) ;
#4761=DIRECTION ( 'NONE',  ( 0.000000000000000000, 0.000000000000000000, 1.000000000000000000 ) ) ;
#4764=CARTESIAN_POINT ( 'NONE',  ( 98.40734512546775647, 23.25070940071369208, 139.1143251403882459 ) ) ;
#4766=ORIENTED_EDGE ( 'NONE', *, *, #3813, .T. ) ;
#4777=CARTESIAN_POINT ( 'NONE',  ( 25.81270058232203013, 0.000000000000000000, 139.1143251403882459 ) ) ;
#4779=ADVANCED_FACE ( 'NONE', ( #2009 ), #12641, .F. ) ;
#4786=VERTEX_POINT ( 'NONE', #2629 ) ;
#4796=DIRECTION ( 'NONE',  ( 0.000000000000000000, 1.000000000000000000, -0.000000000000000000 ) ) ;
#4799=EDGE_CURVE ( 'NONE', #8184, #11541, #105, .T. ) ;
#4810=LINE ( 'NONE', #7040, #4126 ) ;
#4816=VERTEX_POINT ( 'NONE', #4712 ) ;
#4819=ADVANCED_FACE ( 'NONE', ( #254 ), #14338, .T. ) ;
#4834=VERTEX_POINT ( 'NONE', #8262 ) ;
#4843=ORIENTED_EDGE ( 'NONE', *, *, #10333, .F. ) ;
#4857=AXIS2_PLACEMENT_3D ( 'NONE', #9120, #13806, #5511 ) ;
#4859=CARTESIAN_POINT ( 'NONE',  ( 27.55953187330915810, 0.000000000000000000, 33.00000000000012790 ) ) ;
#4860=ORIENTED_EDGE ( 'NONE', *, *, #2083, .F. ) ;
#4864=CARTESIAN_POINT ( 'NONE',  ( 105.5545870572953930, 15.25070940071369563, 13.14990448602692474 ) ) ;
#4869=DIRECTION ( 'NONE',  ( -1.000000000000000000, 0.000000000000000000, 0.000000000000000000 ) ) ;
#4873=LINE ( 'NONE', #10876, #11009 ) ;
#4876=PLANE ( 'NONE',  #8109 ) ;
#4882=CARTESIAN_POINT ( 'NONE',  ( 58.00000000000000711, 23.25070940071368852, -33.00000000000012790 ) ) ;
#4885=EDGE_CURVE ( 'NONE', #587, #8236, #13105, .T. ) ;
#4890=CARTESIAN_POINT ( 'NONE',  ( 0.000000000000000000, 21.75070940071369918, 33.00000000000012790 ) ) ;
#4903=DIRECTION ( 'NONE',  ( 0.000000000000000000, 1.000000000000000000, -0.000000000000000000 ) ) ;
#4904=ORIENTED_EDGE ( 'NONE', *, *, #12171, .T. ) ;
#4910=VECTOR ( 'NONE', #2853, 1000.000000000000000 ) ;
#4917=ORIENTED_EDGE ( 'NONE', *, *, #5015, .T. ) ;
#4920=DIRECTION ( 'NONE',  ( 1.000000000000000000, 1.156482317317870492E-16, 0.000000000000000000 ) ) ;
#4925=CARTESIAN_POINT ( 'NONE',  ( 105.5545870572953930, 23.25070940071369563, 13.14990448602693007 ) ) ;
#4929=LINE ( 'NONE', #2550, #12824 ) ;
#4938=EDGE_LOOP ( 'NONE', ( #14440, #8595, #749, #10706 ) ) ;
#4943=VECTOR ( 'NONE', #12300, 1000.000000000000000 ) ;
#4944=CARTESIAN_POINT ( 'NONE',  ( 112.9262740340969060, 0.000000000000000000, 139.1143251403882459 ) ) ;
#4945=CARTESIAN_POINT ( 'NONE',  ( 50.01091543003727224, 21.75070940071325865, 33.00000000000012790 ) ) ;
#4954=DIRECTION ( 'NONE',  ( -0.000000000000000000, -0.000000000000000000, -1.000000000000000000 ) ) ;
#4955=EDGE_LOOP ( 'NONE', ( #12864, #9914, #10689, #8198 ) ) ;
#4961=CIRCLE ( 'NONE', #13550, 4.000000000000003553 ) ;
#4969=ORIENTED_EDGE ( 'NONE', *, *, #1143, .T. ) ;
#4977=ORIENTED_EDGE ( 'NONE', *, *, #11614, .F. ) ;
#4983=ORIENTED_EDGE ( 'NONE', *, *, #2019, .F. ) ;
#4989=ORIENTED_EDGE ( 'NONE', *, *, #13743, .F. ) ;
#4997=EDGE_CURVE ( 'NONE', #2975, #1446, #5240, .T. ) ;
#5002=ORIENTED_EDGE ( 'NONE', *, *, #9519, .T. ) ;
#5011=ORIENTED_EDGE ( 'NONE', *, *, #11614, .T. ) ;
#5012=VECTOR ( 'NONE', #14132, 1000.000000000000000 ) ;
#5013=DIRECTION ( 'NONE',  ( -1.000000000000000000, 0.000000000000000000, 0.000000000000000000 ) ) ;
#5014=VECTOR ( 'NONE', #12158, 1000.000000000000000 ) ;
#5015=EDGE_CURVE ( 'NONE', #5487, #10906, #3999, .T. ) ;
#5016=VERTEX_POINT ( 'NONE', #10949 ) ;
#5027=CARTESIAN_POINT ( 'NONE',  ( 109.8334623555409735, 0.000000000000000000, 139.1143251403882459 ) ) ;
#5045=UNCERTAINTY_MEASURE_WITH_UNIT (LENGTH_MEASURE( 1.000000000000000082E-05 ), #13903, 'distance_accuracy_value', 'NONE');
#5051=ORIENTED_EDGE ( 'NONE', *, *, #3303, .T. ) ;
#5054=EDGE_CURVE ( 'NONE', #5462, #4285, #1556, .T. ) ;
#5057=ORIENTED_EDGE ( 'NONE', *, *, #6340, .F. ) ;
#5061=VERTEX_POINT ( 'NONE', #14767 ) ;
#5068=VECTOR ( 'NONE', #13927, 1000.000000000000000 ) ;
#5075=ORIENTED_EDGE ( 'NONE', *, *, #14778, .T. ) ;
#5077=DIRECTION ( 'NONE',  ( 0.000000000000000000, 1.000000000000000000, -0.000000000000000000 ) ) ;
#5078=CARTESIAN_POINT ( 'NONE',  ( 48.00000000000000000, -2.664535259100377906E-14, -33.00000000000012790 ) ) ;
#5098=DIRECTION ( 'NONE',  ( 0.000000000000000000, 0.000000000000000000, 1.000000000000000000 ) ) ;
#5099=EDGE_CURVE ( 'NONE', #14376, #4084, #12624, .T. ) ;
#5102=ADVANCED_FACE ( 'NONE', ( #7773 ), #12461, .F. ) ;
#5116=VECTOR ( 'NONE', #13998, 1000.000000000000000 ) ;
#5121=EDGE_CURVE ( 'NONE', #8955, #7944, #9076, .T. ) ;
#5122=ORIENTED_EDGE ( 'NONE', *, *, #7446, .F. ) ;
#5124=CARTESIAN_POINT ( 'NONE',  ( 0.000000000000000000, 21.75070940071322667, 139.1143251403882459 ) ) ;
#5125=ORIENTED_EDGE ( 'NONE', *, *, #12152, .T. ) ;
#5148=AXIS2_PLACEMENT_3D ( 'NONE', #3167, #5405, #3245 ) ;
#5150=CARTESIAN_POINT ( 'NONE',  ( 58.00000000000000711, -2.249290599286311032, 33.00000000000012790 ) ) ;
#5152=DIRECTION ( 'NONE',  ( 0.000000000000000000, 1.000000000000000000, -0.000000000000000000 ) ) ;
#5155=LINE ( 'NONE', #6095, #10281 ) ;
#5157=ORIENTED_EDGE ( 'NONE', *, *, #2651, .F. ) ;
#5164=CARTESIAN_POINT ( 'NONE',  ( -2.016677571526633510E-15, 23.25070940071368497, 33.00000000000012790 ) ) ;
#5166=ADVANCED_FACE ( 'NONE', ( #13850 ), #3305, .F. ) ;
#5167=CARTESIAN_POINT ( 'NONE',  ( 96.00000000000002842, 2.750709400713692965, 33.00000000000012790 ) ) ;
#5168=PLANE ( 'NONE',  #11044 ) ;
#5177=ADVANCED_FACE ( 'NONE', ( #3383 ), #4615, .F. ) ;
#5181=DIRECTION ( 'NONE',  ( 0.000000000000000000, 0.000000000000000000, 1.000000000000000000 ) ) ;
#5189=CARTESIAN_POINT ( 'NONE',  ( 46.91810375148135392, 21.75070940071322667, 33.00000000000012790 ) ) ;
#5191=CARTESIAN_POINT ( 'NONE',  ( 46.91810375148135392, 23.25070940071368852, -33.00000000000012790 ) ) ;
#5192=CARTESIAN_POINT ( 'NONE',  ( 56.59738969056744651, 0.000000000000000000, 33.00000000000012790 ) ) ;
#5193=ORIENTED_EDGE ( 'NONE', *, *, #10022, .T. ) ;
#5195=DIRECTION ( 'NONE',  ( 0.000000000000000000, 0.000000000000000000, 1.000000000000000000 ) ) ;
#5203=AXIS2_PLACEMENT_3D ( 'NONE', #10560, #12797, #2241 ) ;
#5221=VECTOR ( 'NONE', #12720, 1000.000000000000000 ) ;
#5224=ADVANCED_FACE ( 'NONE', ( #6082 ), #2227, .T. ) ;
#5229=LINE ( 'NONE', #9859, #5758 ) ;
#5237=AXIS2_PLACEMENT_3D ( 'NONE', #2852, #4071, #4154 ) ;
#5240=LINE ( 'NONE', #5164, #14792 ) ;
#5244=ORIENTED_EDGE ( 'NONE', *, *, #9422, .T. ) ;
#5252=VERTEX_POINT ( 'NONE', #8080 ) ;
#5274=PLANE ( 'NONE',  #8663 ) ;
#5278=EDGE_CURVE ( 'NONE', #1911, #2542, #15060, .T. ) ;
#5289=DIRECTION ( 'NONE',  ( 0.000000000000000000, 0.000000000000000000, 1.000000000000000000 ) ) ;
#5292=DIRECTION ( 'NONE',  ( -0.000000000000000000, -0.000000000000000000, -1.000000000000000000 ) ) ;
#5293=PLANE ( 'NONE',  #9992 ) ;
#5301=LINE ( 'NONE', #1614, #3039 ) ;
#5303=AXIS2_PLACEMENT_3D ( 'NONE', #12888, #11637, #11316 ) ;
#5304=CARTESIAN_POINT ( 'NONE',  ( 56.59738969056744651, 23.25070940071368852, -33.00000000000012790 ) ) ;
#5309=LINE ( 'NONE', #10007, #14212 ) ;
#5313=VECTOR ( 'NONE', #8095, 1000.000000000000000 ) ;
#5332=DIRECTION ( 'NONE',  ( -0.000000000000000000, -0.000000000000000000, -1.000000000000000000 ) ) ;
#5335=CARTESIAN_POINT ( 'NONE',  ( -2.016677571526633510E-15, 23.25070940071368497, 139.1143251403882459 ) ) ;
#5339=ADVANCED_FACE ( 'NONE', ( #8604 ), #7526, .F. ) ;
#5348=FACE_OUTER_BOUND ( 'NONE', #4955, .T. ) ;
#5353=CLOSED_SHELL ( 'NONE', ( #3849, #14515, #11108, #13304, #7733, #4779, #837, #2287, #5224, #799, #14374, #9773, #3877, #9365, #14127, #5339, #3485, #14029, #8428, #14550, #845, #741, #1830, #1841, #33, #5102, #14027, #7427, #10278, #1053, #1261, #14091, #4269, #14660, #7192, #13655, #8208, #9382, #14360, #13876, #1153, #11806, #10012, #7714, #8569, #3507, #9719, #8216, #14782, #11305, #15163, #12659, #5177, #9796, #12964, #8575, #12774, #9284, #4014, #15025, #11388, #11371, #4819, #14310, #10934, #6432, #8528, #2352, #4520, #9033, #2216, #11460, #11862, #7344, #751, #1280, #573, #5166, #3390, #4335, #3776, #5823, #3259 ) ) ;
#5356=CARTESIAN_POINT ( 'NONE',  ( 118.0000000000000284, 23.25070940071369563, 139.1143251403882459 ) ) ;
#5369=DIRECTION ( 'NONE',  ( -1.000000000000000000, -8.673617379884035472E-17, 0.000000000000000000 ) ) ;
#5380=LINE ( 'NONE', #7766, #2900 ) ;
#5383=VERTEX_POINT ( 'NONE', #13444 ) ;
#5384=EDGE_LOOP ( 'NONE', ( #1467, #10823, #4533, #9827 ) ) ;
#5391=CARTESIAN_POINT ( 'NONE',  ( 103.2469880950108063, 0.000000000000000000, 33.00000000000012790 ) ) ;
#5400=VECTOR ( 'NONE', #8066, 1000.000000000000000 ) ;
#5404=LINE ( 'NONE', #7015, #7913 ) ;
#5405=DIRECTION ( 'NONE',  ( -0.000000000000000000, -0.000000000000000000, -1.000000000000000000 ) ) ;
#5407=LINE ( 'NONE', #12563, #5221 ) ;
#5415=VERTEX_POINT ( 'NONE', #1682 ) ;
#5417=ORIENTED_EDGE ( 'NONE', *, *, #5917, .F. ) ;
#5422=CARTESIAN_POINT ( 'NONE',  ( 58.00000000000000711, 23.25070940071368852, 33.00000000000012790 ) ) ;
#5427=VECTOR ( 'NONE', #3275, 1000.000000000000000 ) ;
#5429=CARTESIAN_POINT ( 'NONE',  ( 30.65234355186507997, 21.75070940071312364, 33.00000000000012790 ) ) ;
#5437=VERTEX_POINT ( 'NONE', #6822 ) ;
#5443=FACE_OUTER_BOUND ( 'NONE', #10242, .T. ) ;
#5450=AXIS2_PLACEMENT_3D ( 'NONE', #5124, #8877, #8721 ) ;
#5455=EDGE_CURVE ( 'NONE', #8958, #1506, #5603, .T. ) ;
#5462=VERTEX_POINT ( 'NONE', #735 ) ;
#5464=ORIENTED_EDGE ( 'NONE', *, *, #1529, .T. ) ;
#5470=EDGE_CURVE ( 'NONE', #11241, #3666, #10214, .T. ) ;
#5486=DIRECTION ( 'NONE',  ( 0.000000000000000000, -0.000000000000000000, 1.000000000000000000 ) ) ;
#5487=VERTEX_POINT ( 'NONE', #7754 ) ;
#5489=DIRECTION ( 'NONE',  ( 1.156482317317870492E-16, -1.000000000000000000, 0.000000000000000000 ) ) ;
#5496=LINE ( 'NONE', #5644, #11247 ) ;
#5500=ORIENTED_EDGE ( 'NONE', *, *, #4716, .F. ) ;
#5511=DIRECTION ( 'NONE',  ( -1.000000000000000000, 0.000000000000000000, 0.000000000000000000 ) ) ;
#5525=EDGE_CURVE ( 'NONE', #13907, #14067, #661, .T. ) ;
#5528=DIRECTION ( 'NONE',  ( 0.000000000000000000, 1.000000000000000000, 0.000000000000000000 ) ) ;
#5539=DIRECTION ( 'NONE',  ( -1.000000000000000000, -8.673617379884035472E-17, 0.000000000000000000 ) ) ;
#5540=ORIENTED_EDGE ( 'NONE', *, *, #1175, .T. ) ;
#5543=CARTESIAN_POINT ( 'NONE',  ( 68.00000000000001421, 1.887379141862766624E-13, 33.00000000000012790 ) ) ;
#5552=EDGE_LOOP ( 'NONE', ( #14003, #2398, #7681, #13218 ) ) ;
#5555=DIRECTION ( 'NONE',  ( -1.000000000000000000, 0.000000000000000000, 0.000000000000000000 ) ) ;
#5557=DIRECTION ( 'NONE',  ( 1.000000000000000000, 0.000000000000000000, 0.000000000000000000 ) ) ;
#5560=DIRECTION ( 'NONE',  ( 1.000000000000000000, -0.000000000000000000, -0.000000000000000000 ) ) ;
#5567=DIRECTION ( 'NONE',  ( 8.673617379884035472E-17, -1.000000000000000000, 0.000000000000000000 ) ) ;
#5598=ORIENTED_EDGE ( 'NONE', *, *, #12380, .T. ) ;
#5600=LINE ( 'NONE', #8137, #11204 ) ;
#5601=VECTOR ( 'NONE', #6289, 1000.000000000000000 ) ;
#5602=PLANE ( 'NONE',  #1144 ) ;
#5603=LINE ( 'NONE', #12678, #2529 ) ;
#5614=VERTEX_POINT ( 'NONE', #1054 ) ;
#5618=ORIENTED_EDGE ( 'NONE', *, *, #7776, .T. ) ;
#5621=EDGE_LOOP ( 'NONE', ( #9369, #4969, #12453, #6927 ) ) ;
#5623=DIRECTION ( 'NONE',  ( 0.000000000000000000, 1.000000000000000000, -0.000000000000000000 ) ) ;
#5626=EDGE_CURVE ( 'NONE', #5719, #14453, #2365, .T. ) ;
#5638=AXIS2_PLACEMENT_3D ( 'NONE', #12550, #3014, #12396 ) ;
#5644=CARTESIAN_POINT ( 'NONE',  ( 0.000000000000000000, 15.25070940071368497, -33.00000000000012790 ) ) ;
#5651=ORIENTED_EDGE ( 'NONE', *, *, #4060, .T. ) ;
#5653=PLANE ( 'NONE',  #970 ) ;
#5662=DIRECTION ( 'NONE',  ( -0.000000000000000000, -0.000000000000000000, -1.000000000000000000 ) ) ;
#5676=ORIENTED_EDGE ( 'NONE', *, *, #6454, .F. ) ;
#5685=CARTESIAN_POINT ( 'NONE',  ( 37.23881781239525424, 23.25070940071368852, 33.00000000000012790 ) ) ;
#5697=VERTEX_POINT ( 'NONE', #10448 ) ;
#5702=EDGE_CURVE ( 'NONE', #14453, #8536, #10393, .T. ) ;
#5706=LINE ( 'NONE', #3078, #10966 ) ;
#5719=VERTEX_POINT ( 'NONE', #4030 ) ;
#5724=EDGE_CURVE ( 'NONE', #11167, #14965, #7442, .T. ) ;
#5729=DIRECTION ( 'NONE',  ( 0.000000000000000000, 1.000000000000000000, -0.000000000000000000 ) ) ;
#5743=LINE ( 'NONE', #5894, #6657 ) ;
#5753=DIRECTION ( 'NONE',  ( 0.000000000000000000, 1.000000000000000000, -0.000000000000000000 ) ) ;
#5758=VECTOR ( 'NONE', #1757, 1000.000000000000000 ) ;
#5759=VERTEX_POINT ( 'NONE', #13356 ) ;
#5761=EDGE_CURVE ( 'NONE', #11670, #7393, #7509, .T. ) ;
#5764=DIRECTION ( 'NONE',  ( 0.000000000000000000, 1.000000000000000000, -0.000000000000000000 ) ) ;
#5781=CARTESIAN_POINT ( 'NONE',  ( 0.000000000000000000, 21.75070940071319114, 33.00000000000012790 ) ) ;
#5782=CARTESIAN_POINT ( 'NONE',  ( 0.000000000000000000, 21.75070940071366365, 139.1143251403882459 ) ) ;
#5794=EDGE_CURVE ( 'NONE', #7261, #13742, #216, .T. ) ;
#5801=LINE ( 'NONE', #10417, #9242 ) ;
#5802=DIRECTION ( 'NONE',  ( 1.000000000000000000, 0.000000000000000000, 0.000000000000000000 ) ) ;
#5814=PLANE ( 'NONE',  #10374 ) ;
#5815=ORIENTED_EDGE ( 'NONE', *, *, #8146, .T. ) ;
#5823=ADVANCED_FACE ( 'NONE', ( #9690 ), #14375, .T. ) ;
#5826=ORIENTED_EDGE ( 'NONE', *, *, #2460, .F. ) ;
#5827=CARTESIAN_POINT ( 'NONE',  ( 112.9262740340969060, 23.25070940071369563, 13.14990448602692474 ) ) ;
#5830=LINE ( 'NONE', #8368, #14764 ) ;
#5840=AXIS2_PLACEMENT_3D ( 'NONE', #370, #299, #8465 ) ;
#5844=FACE_OUTER_BOUND ( 'NONE', #9007, .T. ) ;
#5845=LINE ( 'NONE', #1127, #3882 ) ;
#5846=CARTESIAN_POINT ( 'NONE',  ( -2.688903428702175252E-15, 23.25070940071368142, 139.1143251403882459 ) ) ;
#5853=VECTOR ( 'NONE', #9051, 1000.000000000000000 ) ;
#5881=LINE ( 'NONE', #2326, #1176 ) ;
#5886=EDGE_CURVE ( 'NONE', #11505, #12456, #2485, .T. ) ;
#5887=CARTESIAN_POINT ( 'NONE',  ( 18.00000000000001066, 15.25070940071368497, 139.1143251403882459 ) ) ;
#5894=CARTESIAN_POINT ( 'NONE',  ( -2.016677571526633510E-15, 23.25070940071368497, -33.00000000000012790 ) ) ;
#5898=EDGE_CURVE ( 'NONE', #15116, #9700, #10720, .T. ) ;
#5903=DIRECTION ( 'NONE',  ( -0.000000000000000000, -0.000000000000000000, -1.000000000000000000 ) ) ;
#5911=FACE_OUTER_BOUND ( 'NONE', #14981, .T. ) ;
#5912=ORIENTED_EDGE ( 'NONE', *, *, #3952, .T. ) ;
#5917=EDGE_CURVE ( 'NONE', #5016, #4237, #8346, .T. ) ;
#5918=DIRECTION ( 'NONE',  ( -0.000000000000000000, -0.000000000000000000, -1.000000000000000000 ) ) ;
#5926=DIRECTION ( 'NONE',  ( 1.000000000000000000, 0.000000000000000000, 0.000000000000000000 ) ) ;
#5927=VERTEX_POINT ( 'NONE', #6035 ) ;
#5929=VERTEX_POINT ( 'NONE', #6263 ) ;
#5943=DIRECTION ( 'NONE',  ( 0.000000000000000000, 1.000000000000000000, -0.000000000000000000 ) ) ;
#5949=PLANE ( 'NONE',  #9146 ) ;
#5952=ORIENTED_EDGE ( 'NONE', *, *, #4655, .F. ) ;
#5960=LINE ( 'NONE', #12957, #9802 ) ;
#5968=CARTESIAN_POINT ( 'NONE',  ( 114.6731053250840233, 0.000000000000000000, 139.1143251403882459 ) ) ;
#5973=LINE ( 'NONE', #3721, #1297 ) ;
#5976=VECTOR ( 'NONE', #8491, 1000.000000000000000 ) ;
#5977=LINE ( 'NONE', #1262, #11461 ) ;
#5987=PRODUCT_DEFINITION_CONTEXT ( 'detailed design', #8511, 'design' ) ;
#5995=CARTESIAN_POINT ( 'NONE',  ( 32.39917484285220439, 21.75070940071312364, -33.00000000000012790 ) ) ;
#6002=ORIENTED_EDGE ( 'NONE', *, *, #2019, .T. ) ;
#6003=EDGE_CURVE ( 'NONE', #5415, #11647, #14703, .T. ) ;
#6007=VERTEX_POINT ( 'NONE', #1996 ) ;
#6033=PLANE ( 'NONE',  #12984 ) ;
#6035=CARTESIAN_POINT ( 'NONE',  ( 100.1541764164548880, 23.25070940071369208, 33.00000000000012790 ) ) ;
#6044=DIRECTION ( 'NONE',  ( -1.000000000000000000, -8.673617379884035472E-17, 0.000000000000000000 ) ) ;
#6055=CARTESIAN_POINT ( 'NONE',  ( 108.0866310645538562, 0.000000000000000000, 33.00000000000012790 ) ) ;
#6057=LINE ( 'NONE', #14216, #1263 ) ;
#6060=DIRECTION ( 'NONE',  ( -0.000000000000000000, -0.000000000000000000, -1.000000000000000000 ) ) ;
#6066=CARTESIAN_POINT ( 'NONE',  ( 30.65234355186507997, 0.000000000000000000, 33.00000000000012790 ) ) ;
#6069=EDGE_LOOP ( 'NONE', ( #3184, #3890, #14672, #2203 ) ) ;
#6073=CARTESIAN_POINT ( 'NONE',  ( 0.000000000000000000, 21.75070940071359615, -33.00000000000012790 ) ) ;
#6082=FACE_OUTER_BOUND ( 'NONE', #11170, .T. ) ;
#6085=VECTOR ( 'NONE', #6044, 1000.000000000000000 ) ;
#6089=EDGE_CURVE ( 'NONE', #9571, #13132, #13113, .T. ) ;
#6092=VECTOR ( 'NONE', #6676, 1000.000000000000000 ) ;
#6095=CARTESIAN_POINT ( 'NONE',  ( 103.2469880950108063, 23.25070940071369208, 139.1143251403882459 ) ) ;
#6102=VERTEX_POINT ( 'NONE', #3015 ) ;
#6111=LINE ( 'NONE', #5887, #13966 ) ;
#6121=CARTESIAN_POINT ( 'NONE',  ( 0.000000000000000000, 21.75070940071315562, 139.1143251403882459 ) ) ;
#6123=ORIENTED_EDGE ( 'NONE', *, *, #12887, .T. ) ;
#6125=PLANE ( 'NONE',  #4206 ) ;
#6134=CARTESIAN_POINT ( 'NONE',  ( 104.0000000000000426, 15.25070940071369563, -33.00000000000014211 ) ) ;
#6142=VECTOR ( 'NONE', #11249, 1000.000000000000000 ) ;
#6148=PLANE ( 'NONE',  #8445 ) ;
#6149=LINE ( 'NONE', #368, #2405 ) ;
#6150=AXIS2_PLACEMENT_3D ( 'NONE', #8250, #3549, #14095 ) ;
#6151=VECTOR ( 'NONE', #10039, 1000.000000000000000 ) ;
#6156=ORIENTED_EDGE ( 'NONE', *, *, #7904, .F. ) ;
#6180=ORIENTED_EDGE ( 'NONE', *, *, #2083, .T. ) ;
#6183=CARTESIAN_POINT ( 'NONE',  ( 56.59738969056744651, 23.25070940071368852, 139.1143251403882459 ) ) ;
#6202=LINE ( 'NONE', #11886, #12712 ) ;
#6204=AXIS2_PLACEMENT_3D ( 'NONE', #4570, #10727, #1257 ) ;
#6205=CARTESIAN_POINT ( 'NONE',  ( 98.40734512546775647, 0.000000000000000000, 139.1143251403882459 ) ) ;
#6211=ORIENTED_EDGE ( 'NONE', *, *, #6003, .T. ) ;
#6214=VERTEX_POINT ( 'NONE', #7008 ) ;
#6217=ORIENTED_EDGE ( 'NONE', *, *, #5121, .T. ) ;
#6222=VECTOR ( 'NONE', #12130, 1000.000000000000000 ) ;
#6227=EDGE_CURVE ( 'NONE', #14235, #9917, #8613, .T. ) ;
#6236=ORIENTED_EDGE ( 'NONE', *, *, #7826, .T. ) ;
#6251=ORIENTED_EDGE ( 'NONE', *, *, #2741, .F. ) ;
#6252=AXIS2_PLACEMENT_3D ( 'NONE', #11194, #14658, #12359 ) ;
#6258=DIRECTION ( 'NONE',  ( -1.000000000000000000, -8.673617379884035472E-17, 0.000000000000000000 ) ) ;
#6263=CARTESIAN_POINT ( 'NONE',  ( 18.00000000000001066, 23.25070940071368497, -33.00000000000012790 ) ) ;
#6276=ORIENTED_EDGE ( 'NONE', *, *, #13173, .F. ) ;
#6286=ORIENTED_EDGE ( 'NONE', *, *, #10488, .T. ) ;
#6289=DIRECTION ( 'NONE',  ( 0.000000000000000000, 1.000000000000000000, -0.000000000000000000 ) ) ;
#6290=ORIENTED_EDGE ( 'NONE', *, *, #8077, .F. ) ;
#6292=DIRECTION ( 'NONE',  ( 0.000000000000000000, 1.000000000000000000, -0.000000000000000000 ) ) ;
#6297=VECTOR ( 'NONE', #14924, 1000.000000000000000 ) ;
#6310=DIRECTION ( 'NONE',  ( -0.000000000000000000, -0.000000000000000000, -1.000000000000000000 ) ) ;
#6314=ORIENTED_EDGE ( 'NONE', *, *, #14415, .F. ) ;
#6315=AXIS2_PLACEMENT_3D ( 'NONE', #4082, #8567, #11096 ) ;
#6329=CARTESIAN_POINT ( 'NONE',  ( 130.4454129427046496, -1.749290599286305259, 13.14990448602692474 ) ) ;
#6335=ORIENTED_EDGE ( 'NONE', *, *, #13636, .T. ) ;
#6337=VECTOR ( 'NONE', #6505, 1000.000000000000000 ) ;
#6338=LINE ( 'NONE', #11030, #13210 ) ;
#6340=EDGE_CURVE ( 'NONE', #6102, #5252, #11852, .T. ) ;
#6350=EDGE_LOOP ( 'NONE', ( #4161, #9699, #11896, #15121 ) ) ;
#6351=CARTESIAN_POINT ( 'NONE',  ( 114.0000000000000284, 15.25070940071369563, 139.1143251403882459 ) ) ;
#6356=CARTESIAN_POINT ( 'NONE',  ( 109.8334623555409735, 21.75070940071366365, 33.00000000000012790 ) ) ;
#6361=CARTESIAN_POINT ( 'NONE',  ( -16.99999999999998579, -2.249290599286303927, 33.00000000000012790 ) ) ;
#6364=DIRECTION ( 'NONE',  ( 0.000000000000000000, -0.000000000000000000, -1.000000000000000000 ) ) ;
#6377=CIRCLE ( 'NONE', #9326, 4.000000000000003553 ) ;
#6388=SHAPE_DEFINITION_REPRESENTATION ( #4375, #13539 ) ;
#6393=PLANE ( 'NONE',  #558 ) ;
#6400=ORIENTED_EDGE ( 'NONE', *, *, #10279, .F. ) ;
#6401=CARTESIAN_POINT ( 'NONE',  ( 58.00000000000000711, -2.249290599286311032, -33.00000000000012790 ) ) ;
#6415=ORIENTED_EDGE ( 'NONE', *, *, #12965, .F. ) ;
#6419=FACE_OUTER_BOUND ( 'NONE', #3885, .T. ) ;
#6432=ADVANCED_FACE ( 'NONE', ( #8755 ), #6456, .F. ) ;
#6433=LINE ( 'NONE', #8892, #6337 ) ;
#6434=AXIS2_PLACEMENT_3D ( 'NONE', #4777, #12938, #14164 ) ;
#6443=FACE_OUTER_BOUND ( 'NONE', #1190, .T. ) ;
#6449=ORIENTED_EDGE ( 'NONE', *, *, #10446, .F. ) ;
#6454=EDGE_CURVE ( 'NONE', #14376, #8736, #13380, .T. ) ;
#6456=PLANE ( 'NONE',  #2045 ) ;
#6459=DIRECTION ( 'NONE',  ( 0.000000000000000000, -0.000000000000000000, 1.000000000000000000 ) ) ;
#6460=VERTEX_POINT ( 'NONE', #600 ) ;
#6478=ORIENTED_EDGE ( 'NONE', *, *, #10794, .F. ) ;
#6484=CARTESIAN_POINT ( 'NONE',  ( 100.1541764164548880, 21.75070940071359615, -33.00000000000012790 ) ) ;
#6485=ORIENTED_EDGE ( 'NONE', *, *, #9661, .F. ) ;
#6486=LINE ( 'NONE', #626, #11426 ) ;
#6487=EDGE_CURVE ( 'NONE', #9446, #11132, #12381, .T. ) ;
#6493=ORIENTED_EDGE ( 'NONE', *, *, #11876, .F. ) ;
#6494=EDGE_CURVE ( 'NONE', #8958, #13411, #11067, .T. ) ;
#6499=CARTESIAN_POINT ( 'NONE',  ( 56.59738969056744651, 21.75070940071329417, 139.1143251403882459 ) ) ;
#6500=LINE ( 'NONE', #577, #2122 ) ;
#6503=CARTESIAN_POINT ( 'NONE',  ( 108.0866310645538562, 0.000000000000000000, 139.1143251403882459 ) ) ;
#6504=LINE ( 'NONE', #11125, #14355 ) ;
#6505=DIRECTION ( 'NONE',  ( -0.000000000000000000, -0.000000000000000000, -1.000000000000000000 ) ) ;
#6510=ORIENTED_EDGE ( 'NONE', *, *, #4385, .T. ) ;
#6513=DIRECTION ( 'NONE',  ( 0.000000000000000000, 0.000000000000000000, 1.000000000000000000 ) ) ;
#6518=EDGE_LOOP ( 'NONE', ( #3101, #14958, #12191, #14628, #3459, #6536, #10674, #8089, #11315, #14858, #12534, #12922, #2873, #3373, #94, #11910, #4766, #7516, #10182, #5598, #9603, #15081, #14539, #4100, #2472, #1137, #11464, #4687, #7703, #9324, #7694, #12186, #9765, #2960, #6156, #12494, #2627, #6449, #13989, #4977, #13691, #1394, #15153, #1972, #6123, #3458, #6938, #9752, #5651, #7572, #5500, #12298, #8464, #8875, #5676, #3824, #8310, #9402, #13614, #4713, #5125, #14457, #6251, #6236, #14598, #14100 ) ) ;
#6526=ORIENTED_EDGE ( 'NONE', *, *, #1346, .F. ) ;
#6527=ORIENTED_EDGE ( 'NONE', *, *, #2123, .T. ) ;
#6531=DIRECTION ( 'NONE',  ( 1.156482317317870492E-16, -1.000000000000000000, 0.000000000000000000 ) ) ;
#6532=EDGE_CURVE ( 'NONE', #5487, #9598, #7470, .T. ) ;
#6533=EDGE_CURVE ( 'NONE', #5927, #1834, #5229, .T. ) ;
#6536=ORIENTED_EDGE ( 'NONE', *, *, #2501, .T. ) ;
#6545=EDGE_LOOP ( 'NONE', ( #7428, #11083, #2120, #5417 ) ) ;
#6548=EDGE_CURVE ( 'NONE', #11623, #6609, #5301, .T. ) ;
#6559=VECTOR ( 'NONE', #9458, 1000.000000000000000 ) ;
#6562=CIRCLE ( 'NONE', #14449, 4.000000000000003553 ) ;
#6564=DIRECTION ( 'NONE',  ( -1.000000000000000000, -1.156482317317870492E-16, 0.000000000000000000 ) ) ;
#6565=CARTESIAN_POINT ( 'NONE',  ( 32.39917484285220439, 23.25070940071368852, 33.00000000000012790 ) ) ;
#6567=VERTEX_POINT ( 'NONE', #4526 ) ;
#6594=EDGE_CURVE ( 'NONE', #4084, #13411, #4602, .T. ) ;
#6598=EDGE_CURVE ( 'NONE', #2975, #3404, #4681, .T. ) ;
#6609=VERTEX_POINT ( 'NONE', #12612 ) ;
#6611=DIRECTION ( 'NONE',  ( 1.000000000000000000, 1.156482317317870492E-16, 0.000000000000000000 ) ) ;
#6618=CARTESIAN_POINT ( 'NONE',  ( -2.016677571526633510E-15, 23.25070940071368497, 139.1143251403882459 ) ) ;
#6630=CARTESIAN_POINT ( 'NONE',  ( 0.000000000000000000, 21.75070940071312364, -33.00000000000012790 ) ) ;
#6631=ORIENTED_EDGE ( 'NONE', *, *, #2232, .T. ) ;
#6633=AXIS2_PLACEMENT_3D ( 'NONE', #1926, #5555, #8014 ) ;
#6657=VECTOR ( 'NONE', #11799, 1000.000000000000000 ) ;
#6663=DIRECTION ( 'NONE',  ( -1.000000000000000000, 0.000000000000000000, 0.000000000000000000 ) ) ;
#6668=VECTOR ( 'NONE', #9684, 1000.000000000000000 ) ;
#6673=CARTESIAN_POINT ( 'NONE',  ( 104.0000000000000426, 11.25070940071369563, 139.1143251403882459 ) ) ;
#6675=CARTESIAN_POINT ( 'NONE',  ( 130.4454129427046496, 23.25070940071369563, -13.14990448602692474 ) ) ;
#6676=DIRECTION ( 'NONE',  ( -0.000000000000000000, -0.000000000000000000, -1.000000000000000000 ) ) ;
#6683=ORIENTED_EDGE ( 'NONE', *, *, #11959, .F. ) ;
#6685=EDGE_CURVE ( 'NONE', #4816, #14721, #6149, .T. ) ;
#6694=VECTOR ( 'NONE', #14510, 1000.000000000000000 ) ;
#6698=EDGE_LOOP ( 'NONE', ( #10226, #8833, #8288, #8365 ) ) ;
#6701=DIRECTION ( 'NONE',  ( -0.000000000000000000, -0.000000000000000000, -1.000000000000000000 ) ) ;
#6702=ORIENTED_EDGE ( 'NONE', *, *, #7259, .F. ) ;
#6703=CARTESIAN_POINT ( 'NONE',  ( 104.9938193859979236, 21.75070940071363168, 33.00000000000012790 ) ) ;
#6712=EDGE_CURVE ( 'NONE', #4816, #13146, #1444, .T. ) ;
#6717=PLANE ( 'NONE',  #13796 ) ;
#6722=CARTESIAN_POINT ( 'NONE',  ( 95.31453344691183815, 0.000000000000000000, -33.00000000000012790 ) ) ;
#6723=VECTOR ( 'NONE', #5369, 1000.000000000000000 ) ;
#6728=CARTESIAN_POINT ( 'NONE',  ( 100.1541764164548880, 0.000000000000000000, -33.00000000000012790 ) ) ;
#6730=CARTESIAN_POINT ( 'NONE',  ( 30.65234355186507997, 23.25070940071368852, 139.1143251403882459 ) ) ;
#6732=CARTESIAN_POINT ( 'NONE',  ( 109.8334623555409735, 0.000000000000000000, 33.00000000000012790 ) ) ;
#6735=ORIENTED_EDGE ( 'NONE', *, *, #7308, .T. ) ;
#6745=CARTESIAN_POINT ( 'NONE',  ( 88.00000000000002842, 9.769962616701380080E-14, 33.00000000000012790 ) ) ;
#6775=LINE ( 'NONE', #10175, #1958 ) ;
#6782=LINE ( 'NONE', #11395, #3017 ) ;
#6791=VECTOR ( 'NONE', #5662, 1000.000000000000000 ) ;
#6792=VERTEX_POINT ( 'NONE', #9977 ) ;
#6798=FACE_OUTER_BOUND ( 'NONE', #10210, .T. ) ;
#6808=VECTOR ( 'NONE', #3665, 1000.000000000000000 ) ;
#6819=ORIENTED_EDGE ( 'NONE', *, *, #3873, .T. ) ;
#6820=DIRECTION ( 'NONE',  ( 1.000000000000000000, 8.673617379884035472E-17, 0.000000000000000000 ) ) ;
#6822=CARTESIAN_POINT ( 'NONE',  ( 95.31453344691183815, 23.25070940071369208, -33.00000000000012790 ) ) ;
#6826=ORIENTED_EDGE ( 'NONE', *, *, #4060, .F. ) ;
#6829=DIRECTION ( 'NONE',  ( -0.000000000000000000, -0.000000000000000000, -1.000000000000000000 ) ) ;
#6831=ORIENTED_EDGE ( 'NONE', *, *, #3303, .F. ) ;
#6852=PLANE ( 'NONE',  #8120 ) ;
#6853=EDGE_CURVE ( 'NONE', #5462, #8536, #6433, .T. ) ;
#6861=DIRECTION ( 'NONE',  ( 0.000000000000000000, 1.000000000000000000, -0.000000000000000000 ) ) ;
#6863=PLANE ( 'NONE',  #14157 ) ;
#6864=CARTESIAN_POINT ( 'NONE',  ( 0.000000000000000000, 0.000000000000000000, -33.00000000000012790 ) ) ;
#6865=LINE ( 'NONE', #782, #2659 ) ;
#6866=CARTESIAN_POINT ( 'NONE',  ( 100.0000000000000284, 11.25070940071369563, 33.00000000000012790 ) ) ;
#6874=AXIS2_PLACEMENT_3D ( 'NONE', #7250, #12014, #13177 ) ;
#6876=ORIENTED_EDGE ( 'NONE', *, *, #11805, .T. ) ;
#6881=LINE ( 'NONE', #2191, #4087 ) ;
#6882=EDGE_CURVE ( 'NONE', #1679, #13146, #4187, .T. ) ;
#6888=DIRECTION ( 'NONE',  ( -1.156482317317870492E-16, 1.000000000000000000, -0.000000000000000000 ) ) ;
#6891=ORIENTED_EDGE ( 'NONE', *, *, #8572, .T. ) ;
#6903=ORIENTED_EDGE ( 'NONE', *, *, #15074, .T. ) ;
#6910=VERTEX_POINT ( 'NONE', #8592 ) ;
#6915=ORIENTED_EDGE ( 'NONE', *, *, #11959, .T. ) ;
#6916=LINE ( 'NONE', #13688, #12077 ) ;
#6917=ORIENTED_EDGE ( 'NONE', *, *, #9956, .T. ) ;
#6918=ORIENTED_EDGE ( 'NONE', *, *, #9835, .F. ) ;
#6919=VECTOR ( 'NONE', #10442, 1000.000000000000000 ) ;
#6925=LINE ( 'NONE', #9884, #4467 ) ;
#6927=ORIENTED_EDGE ( 'NONE', *, *, #9809, .F. ) ;
#6928=EDGE_CURVE ( 'NONE', #8234, #8468, #11126, .T. ) ;
#6929=DIRECTION ( 'NONE',  ( -0.000000000000000000, -0.000000000000000000, -1.000000000000000000 ) ) ;
#6935=DIRECTION ( 'NONE',  ( -0.000000000000000000, -0.000000000000000000, -1.000000000000000000 ) ) ;
#6938=ORIENTED_EDGE ( 'NONE', *, *, #6882, .F. ) ;
#6944=CARTESIAN_POINT ( 'NONE',  ( 93.56770215592470663, 23.25070940071369208, -33.00000000000012790 ) ) ;
#6953=VECTOR ( 'NONE', #13330, 1000.000000000000000 ) ;
#6961=DIRECTION ( 'NONE',  ( 0.000000000000000000, 0.000000000000000000, 1.000000000000000000 ) ) ;
#6976=EDGE_CURVE ( 'NONE', #4729, #10905, #15131, .T. ) ;
#6979=CARTESIAN_POINT ( 'NONE',  ( 100.0000000000000284, 6.750709400713692965, 33.00000000000012790 ) ) ;
#6981=DIRECTION ( 'NONE',  ( -1.000000000000000000, -8.673617379884035472E-17, 0.000000000000000000 ) ) ;
#6982=EDGE_LOOP ( 'NONE', ( #9380, #11074, #4292, #11931 ) ) ;
#6984=DIRECTION ( 'NONE',  ( -0.000000000000000000, -0.000000000000000000, -1.000000000000000000 ) ) ;
#6993=ORIENTED_EDGE ( 'NONE', *, *, #5626, .F. ) ;
#7008=CARTESIAN_POINT ( 'NONE',  ( 45.17127246049422240, 23.25070940071368852, 33.00000000000012790 ) ) ;
#7011=CARTESIAN_POINT ( 'NONE',  ( 50.01091543003727224, 21.75070940071325865, 139.1143251403882459 ) ) ;
#7015=CARTESIAN_POINT ( 'NONE',  ( 118.0000000000000568, 2.046973701652633381E-13, 33.00000000000012790 ) ) ;
#7028=ORIENTED_EDGE ( 'NONE', *, *, #335, .T. ) ;
#7031=CARTESIAN_POINT ( 'NONE',  ( 104.9938193859979236, 23.25070940071369208, 139.1143251403882459 ) ) ;
#7034=PLANE ( 'NONE',  #7658 ) ;
#7035=CARTESIAN_POINT ( 'NONE',  ( 42.07846078193830408, 0.000000000000000000, 139.1143251403882459 ) ) ;
#7040=CARTESIAN_POINT ( 'NONE',  ( 32.39917484285220439, 23.25070940071368852, 139.1143251403882459 ) ) ;
#7048=ORIENTED_EDGE ( 'NONE', *, *, #7721, .T. ) ;
#7050=VECTOR ( 'NONE', #13081, 1000.000000000000000 ) ;
#7068=EDGE_CURVE ( 'NONE', #12778, #844, #4345, .T. ) ;
#7075=VECTOR ( 'NONE', #1670, 1000.000000000000000 ) ;
#7080=VECTOR ( 'NONE', #9102, 1000.000000000000000 ) ;
#7082=DIRECTION ( 'NONE',  ( 1.000000000000000000, 0.000000000000000000, 0.000000000000000000 ) ) ;
#7083=EDGE_CURVE ( 'NONE', #4346, #1838, #3196, .T. ) ;
#7090=LINE ( 'NONE', #161, #9383 ) ;
#7103=DIRECTION ( 'NONE',  ( -1.000000000000000000, 0.000000000000000000, 0.000000000000000000 ) ) ;
#7106=EDGE_CURVE ( 'NONE', #9234, #8992, #10287, .T. ) ;
#7111=ORIENTED_EDGE ( 'NONE', *, *, #6712, .T. ) ;
#7115=DIRECTION ( 'NONE',  ( 0.000000000000000000, 0.000000000000000000, 1.000000000000000000 ) ) ;
#7116=DIRECTION ( 'NONE',  ( -0.000000000000000000, -0.000000000000000000, -1.000000000000000000 ) ) ;
#7120=VECTOR ( 'NONE', #1629, 1000.000000000000000 ) ;
#7133=ORIENTED_EDGE ( 'NONE', *, *, #6487, .T. ) ;
#7134=VERTEX_POINT ( 'NONE', #11239 ) ;
#7143=VERTEX_POINT ( 'NONE', #8777 ) ;
#7144=PLANE ( 'NONE',  #5840 ) ;
#7145=ORIENTED_EDGE ( 'NONE', *, *, #3568, .F. ) ;
#7157=ORIENTED_EDGE ( 'NONE', *, *, #8646, .F. ) ;
#7163=CARTESIAN_POINT ( 'NONE',  ( 58.00000000000000711, -2.249290599286311032, 139.1143251403882459 ) ) ;
#7169=EDGE_LOOP ( 'NONE', ( #5057, #11744, #2231, #12024 ) ) ;
#7175=DIRECTION ( 'NONE',  ( 1.000000000000000000, 1.156482317317870492E-16, 0.000000000000000000 ) ) ;
#7177=DIRECTION ( 'NONE',  ( 0.000000000000000000, 0.000000000000000000, 1.000000000000000000 ) ) ;
#7183=DIRECTION ( 'NONE',  ( 1.000000000000000000, 0.000000000000000000, 0.000000000000000000 ) ) ;
#7184=ORIENTED_EDGE ( 'NONE', *, *, #6003, .F. ) ;
#7189=PLANE ( 'NONE',  #13827 ) ;
#7192=ADVANCED_FACE ( 'NONE', ( #10174 ), #12325, .T. ) ;
#7194=DIRECTION ( 'NONE',  ( -1.000000000000000000, -1.156482317317871478E-16, 0.000000000000000000 ) ) ;
#7222=ORIENTED_EDGE ( 'NONE', *, *, #7333, .F. ) ;
#7230=ORIENTED_EDGE ( 'NONE', *, *, #13831, .F. ) ;
#7231=LINE ( 'NONE', #8474, #4721 ) ;
#7234=DIRECTION ( 'NONE',  ( -1.000000000000000000, -1.156482317317870492E-16, 0.000000000000000000 ) ) ;
#7241=PLANE ( 'NONE',  #7443 ) ;
#7247=DIRECTION ( 'NONE',  ( -1.000000000000000000, 0.000000000000000000, 0.000000000000000000 ) ) ;
#7250=CARTESIAN_POINT ( 'NONE',  ( -2.688903428702175252E-15, 23.25070940071368142, 139.1143251403882459 ) ) ;
#7253=EDGE_CURVE ( 'NONE', #5759, #7134, #11538, .T. ) ;
#7257=FACE_OUTER_BOUND ( 'NONE', #9863, .T. ) ;
#7259=EDGE_CURVE ( 'NONE', #6007, #7276, #3473, .T. ) ;
#7261=VERTEX_POINT ( 'NONE', #7941 ) ;
#7264=PLANE ( 'NONE',  #2392 ) ;
#7269=CARTESIAN_POINT ( 'NONE',  ( 68.00000000000001421, 1.887379141862766624E-13, -33.00000000000012790 ) ) ;
#7276=VERTEX_POINT ( 'NONE', #15170 ) ;
#7282=LINE ( 'NONE', #9755, #9010 ) ;
#7284=EDGE_CURVE ( 'NONE', #1809, #7515, #13, .T. ) ;
#7286=CARTESIAN_POINT ( 'NONE',  ( -2.016677571526633510E-15, 23.25070940071368497, -33.00000000000012790 ) ) ;
#7294=DIRECTION ( 'NONE',  ( -1.000000000000000000, -8.673617379884035472E-17, 0.000000000000000000 ) ) ;
#7308=EDGE_CURVE ( 'NONE', #6214, #10074, #2620, .T. ) ;
#7309=CARTESIAN_POINT ( 'NONE',  ( 42.07846078193830408, 0.000000000000000000, -33.00000000000012790 ) ) ;
#7314=DIRECTION ( 'NONE',  ( -0.000000000000000000, -0.000000000000000000, -1.000000000000000000 ) ) ;
#7329=DIRECTION ( 'NONE',  ( 0.000000000000000000, 1.000000000000000000, 0.000000000000000000 ) ) ;
#7333=EDGE_CURVE ( 'NONE', #4396, #8798, #5155, .T. ) ;
#7334=DIRECTION ( 'NONE',  ( -1.000000000000000000, -1.156482317317870492E-16, 0.000000000000000000 ) ) ;
#7343=CARTESIAN_POINT ( 'NONE',  ( 104.9938193859979236, 23.25070940071369208, -33.00000000000012790 ) ) ;
#7344=ADVANCED_FACE ( 'NONE', ( #10785 ), #10859, .F. ) ;
#7353=ORIENTED_EDGE ( 'NONE', *, *, #1143, .F. ) ;
#7359=CARTESIAN_POINT ( 'NONE',  ( 50.01091543003727224, 0.000000000000000000, 139.1143251403882459 ) ) ;
#7364=DIRECTION ( 'NONE',  ( 0.000000000000000000, 0.000000000000000000, -1.000000000000000000 ) ) ;
#7367=LINE ( 'NONE', #7286, #1312 ) ;
#7370=VECTOR ( 'NONE', #4954, 1000.000000000000000 ) ;
#7379=AXIS2_PLACEMENT_3D ( 'NONE', #4639, #7103, #108 ) ;
#7393=VERTEX_POINT ( 'NONE', #11152 ) ;
#7396=VERTEX_POINT ( 'NONE', #2840 ) ;
#7397=CARTESIAN_POINT ( 'NONE',  ( 68.00000000000000000, 2.750709400713692965, 139.1143251403882459 ) ) ;
#7406=DIRECTION ( 'NONE',  ( 0.000000000000000000, 1.000000000000000000, -0.000000000000000000 ) ) ;
#7415=DIRECTION ( 'NONE',  ( 1.000000000000000000, 0.000000000000000000, 0.000000000000000000 ) ) ;
#7427=ADVANCED_FACE ( 'NONE', ( #1760 ), #3145, .T. ) ;
#7428=ORIENTED_EDGE ( 'NONE', *, *, #10960, .F. ) ;
#7438=LINE ( 'NONE', #13417, #6222 ) ;
#7442=LINE ( 'NONE', #1438, #560 ) ;
#7443=AXIS2_PLACEMENT_3D ( 'NONE', #11929, #8552, #13252 ) ;
#7446=EDGE_CURVE ( 'NONE', #8969, #1527, #5380, .T. ) ;
#7448=DIRECTION ( 'NONE',  ( -1.000000000000000000, -8.673617379884035472E-17, 0.000000000000000000 ) ) ;
#7451=VERTEX_POINT ( 'NONE', #12229 ) ;
#7452=ORIENTED_EDGE ( 'NONE', *, *, #14436, .F. ) ;
#7458=ORIENTED_EDGE ( 'NONE', *, *, #6712, .F. ) ;
#7462=CARTESIAN_POINT ( 'NONE',  ( -2.016677571526633510E-15, 23.25070940071368497, 139.1143251403882459 ) ) ;
#7465=VECTOR ( 'NONE', #1833, 1000.000000000000000 ) ;
#7467=VERTEX_POINT ( 'NONE', #5304 ) ;
#7470=LINE ( 'NONE', #14837, #5014 ) ;
#7486=EDGE_CURVE ( 'NONE', #8402, #4620, #9861, .T. ) ;
#7501=DIRECTION ( 'NONE',  ( 0.000000000000000000, 0.000000000000000000, 1.000000000000000000 ) ) ;
#7503=CARTESIAN_POINT ( 'NONE',  ( 0.000000000000000000, 21.75070940071309167, -33.00000000000012790 ) ) ;
#7507=DIRECTION ( 'NONE',  ( -1.000000000000000000, 0.000000000000000000, 0.000000000000000000 ) ) ;
#7509=LINE ( 'NONE', #2816, #8447 ) ;
#7515=VERTEX_POINT ( 'NONE', #2918 ) ;
#7516=ORIENTED_EDGE ( 'NONE', *, *, #1175, .F. ) ;
#7524=ORIENTED_EDGE ( 'NONE', *, *, #6976, .T. ) ;
#7525=FACE_OUTER_BOUND ( 'NONE', #13703, .T. ) ;
#7526=PLANE ( 'NONE',  #11859 ) ;
#7528=CARTESIAN_POINT ( 'NONE',  ( 27.55953187330915810, 21.75070940071309167, -33.00000000000012790 ) ) ;
#7529=ORIENTED_EDGE ( 'NONE', *, *, #2174, .F. ) ;
#7534=CARTESIAN_POINT ( 'NONE',  ( 109.8334623555409735, 21.75070940071366365, 13.14990448602693007 ) ) ;
#7536=ORIENTED_EDGE ( 'NONE', *, *, #11367, .F. ) ;
#7543=VECTOR ( 'NONE', #2498, 1000.000000000000000 ) ;
#7551=VECTOR ( 'NONE', #11502, 1000.000000000000000 ) ;
#7554=DIRECTION ( 'NONE',  ( -1.156482317317870492E-16, 1.000000000000000000, -0.000000000000000000 ) ) ;
#7567=EDGE_CURVE ( 'NONE', #5252, #13534, #11440, .T. ) ;
#7572=ORIENTED_EDGE ( 'NONE', *, *, #11198, .F. ) ;
#7574=ORIENTED_EDGE ( 'NONE', *, *, #12675, .T. ) ;
#7575=CARTESIAN_POINT ( 'NONE',  ( 114.6731053250840233, 23.25070940071369563, 139.1143251403882459 ) ) ;
#7594=ORIENTED_EDGE ( 'NONE', *, *, #9956, .F. ) ;
#7597=ORIENTED_EDGE ( 'NONE', *, *, #12152, .F. ) ;
#7604=ORIENTED_EDGE ( 'NONE', *, *, #6227, .F. ) ;
#7610=CARTESIAN_POINT ( 'NONE',  ( 0.000000000000000000, 21.75070940071322667, -33.00000000000012790 ) ) ;
#7616=EDGE_LOOP ( 'NONE', ( #6831, #9934, #14838, #6683 ) ) ;
#7618=DIRECTION ( 'NONE',  ( 0.000000000000000000, 1.000000000000000000, 0.000000000000000000 ) ) ;
#7619=EDGE_CURVE ( 'NONE', #9598, #2535, #2066, .T. ) ;
#7622=DIRECTION ( 'NONE',  ( 1.000000000000000000, 0.000000000000000000, 0.000000000000000000 ) ) ;
#7625=CARTESIAN_POINT ( 'NONE',  ( 51.75774672102440377, 0.000000000000000000, 33.00000000000012790 ) ) ;
#7627=CARTESIAN_POINT ( 'NONE',  ( 51.75774672102440377, 0.000000000000000000, -33.00000000000012790 ) ) ;
#7635=PLANE ( 'NONE',  #982 ) ;
#7638=DIRECTION ( 'NONE',  ( 1.000000000000000000, 8.673617379884035472E-17, 0.000000000000000000 ) ) ;
#7639=EDGE_CURVE ( 'NONE', #5697, #8736, #11683, .T. ) ;
#7650=VECTOR ( 'NONE', #2616, 1000.000000000000000 ) ;
#7655=DIRECTION ( 'NONE',  ( -0.000000000000000000, -0.000000000000000000, -1.000000000000000000 ) ) ;
#7658=AXIS2_PLACEMENT_3D ( 'NONE', #10580, #11563, #9429 ) ;
#7666=AXIS2_PLACEMENT_3D ( 'NONE', #12653, #10345, #6961 ) ;
#7676=CARTESIAN_POINT ( 'NONE',  ( 56.59738969056744651, 0.000000000000000000, -33.00000000000012790 ) ) ;
#7681=ORIENTED_EDGE ( 'NONE', *, *, #11876, .T. ) ;
#7689=CARTESIAN_POINT ( 'NONE',  ( 108.0866310645538562, 0.000000000000000000, -33.00000000000012790 ) ) ;
#7693=ORIENTED_EDGE ( 'NONE', *, *, #13636, .F. ) ;
#7694=ORIENTED_EDGE ( 'NONE', *, *, #1883, .F. ) ;
#7695=AXIS2_PLACEMENT_3D ( 'NONE', #5846, #10682, #973 ) ;
#7699=DIRECTION ( 'NONE',  ( -1.000000000000000000, 0.000000000000000000, 0.000000000000000000 ) ) ;
#7700=CARTESIAN_POINT ( 'NONE',  ( 112.9262740340969060, 0.000000000000000000, 13.14990448602693007 ) ) ;
#7703=ORIENTED_EDGE ( 'NONE', *, *, #5794, .T. ) ;
#7705=CIRCLE ( 'NONE', #6252, 9.999999999999994671 ) ;
#7709=CARTESIAN_POINT ( 'NONE',  ( 105.5545870572953930, -1.749290599286305259, -13.14990448602692474 ) ) ;
#7714=ADVANCED_FACE ( 'NONE', ( #14455 ), #7144, .T. ) ;
#7721=EDGE_CURVE ( 'NONE', #3968, #5929, #8529, .T. ) ;
#7733=ADVANCED_FACE ( 'NONE', ( #8597 ), #75, .T. ) ;
#7742=LINE ( 'NONE', #13739, #344 ) ;
#7743=CARTESIAN_POINT ( 'NONE',  ( 98.40734512546775647, 0.000000000000000000, -33.00000000000012790 ) ) ;
#7753=FACE_OUTER_BOUND ( 'NONE', #10917, .T. ) ;
#7754=CARTESIAN_POINT ( 'NONE',  ( 54.85055839958032209, 21.75070940071329417, 33.00000000000012790 ) ) ;
#7758=EDGE_CURVE ( 'NONE', #1679, #10618, #2452, .T. ) ;
#7764=ORIENTED_EDGE ( 'NONE', *, *, #5724, .T. ) ;
#7766=CARTESIAN_POINT ( 'NONE',  ( 40.33162949095117966, 23.25070940071368852, 139.1143251403882459 ) ) ;
#7773=FACE_OUTER_BOUND ( 'NONE', #9683, .T. ) ;
#7774=EDGE_CURVE ( 'NONE', #65, #1549, #9618, .T. ) ;
#7776=EDGE_CURVE ( 'NONE', #1527, #9198, #13148, .T. ) ;
#7792=DIRECTION ( 'NONE',  ( 0.000000000000000000, 1.000000000000000000, -0.000000000000000000 ) ) ;
#7801=VECTOR ( 'NONE', #11892, 1000.000000000000000 ) ;
#7807=DIRECTION ( 'NONE',  ( 1.000000000000000000, -0.000000000000000000, -0.000000000000000000 ) ) ;
#7822=CARTESIAN_POINT ( 'NONE',  ( 51.75774672102440377, 23.25070940071368852, 33.00000000000012790 ) ) ;
#7823=CARTESIAN_POINT ( 'NONE',  ( -2.688903428702175252E-15, 23.25070940071368142, -33.00000000000012790 ) ) ;
#7824=EDGE_CURVE ( 'NONE', #10905, #5061, #12364, .T. ) ;
#7826=EDGE_CURVE ( 'NONE', #1838, #4786, #3621, .T. ) ;
#7831=LINE ( 'NONE', #7676, #270 ) ;
#7855=LINE ( 'NONE', #2073, #6297 ) ;
#7859=DIRECTION ( 'NONE',  ( 0.000000000000000000, -0.000000000000000000, 1.000000000000000000 ) ) ;
#7860=PLANE ( 'NONE',  #5638 ) ;
#7877=DIRECTION ( 'NONE',  ( -1.000000000000000000, -2.775557561562891351E-15, 0.000000000000000000 ) ) ;
#7886=DIRECTION ( 'NONE',  ( 0.000000000000000000, 1.000000000000000000, -0.000000000000000000 ) ) ;
#7892=CARTESIAN_POINT ( 'NONE',  ( 54.00000000000000711, -2.249290599286311032, -33.00000000000012790 ) ) ;
#7895=CARTESIAN_POINT ( 'NONE',  ( 118.0000000000000284, 19.25070940071370273, 139.1143251403882459 ) ) ;
#7898=AXIS2_PLACEMENT_3D ( 'NONE', #2261, #8353, #9586 ) ;
#7899=EDGE_LOOP ( 'NONE', ( #13644, #10077, #6002, #13497 ) ) ;
#7901=CIRCLE ( 'NONE', #9138, 4.000000000000003553 ) ;
#7903=CARTESIAN_POINT ( 'NONE',  ( -2.016677571526633510E-15, 23.25070940071368497, 33.00000000000012790 ) ) ;
#7904=EDGE_CURVE ( 'NONE', #9598, #3404, #3123, .T. ) ;
#7912=EDGE_CURVE ( 'NONE', #14241, #4729, #8130, .T. ) ;
#7913=VECTOR ( 'NONE', #8254, 1000.000000000000000 ) ;
#7928=VECTOR ( 'NONE', #12690, 1000.000000000000000 ) ;
#7929=PLANE ( 'NONE',  #8028 ) ;
#7931=AXIS2_PLACEMENT_3D ( 'NONE', #5782, #10696, #3541 ) ;
#7941=CARTESIAN_POINT ( 'NONE',  ( 46.91810375148135392, 21.75070940071322667, -33.00000000000012790 ) ) ;
#7944=VERTEX_POINT ( 'NONE', #5827 ) ;
#7945=CARTESIAN_POINT ( 'NONE',  ( 0.000000000000000000, 21.75070940071325865, 33.00000000000012790 ) ) ;
#7946=DIRECTION ( 'NONE',  ( 0.000000000000000000, 1.000000000000000000, 0.000000000000000000 ) ) ;
#7950=ORIENTED_EDGE ( 'NONE', *, *, #8077, .T. ) ;
#7953=VECTOR ( 'NONE', #5943, 1000.000000000000000 ) ;
#7960=ORIENTED_EDGE ( 'NONE', *, *, #14118, .T. ) ;
#7964=CARTESIAN_POINT ( 'NONE',  ( 96.00000000000002842, 2.750709400713692965, -33.00000000000012790 ) ) ;
#7968=CARTESIAN_POINT ( 'NONE',  ( 103.2469880950108063, 0.000000000000000000, 139.1143251403882459 ) ) ;
#7969=DIRECTION ( 'NONE',  ( -0.000000000000000000, -0.000000000000000000, -1.000000000000000000 ) ) ;
#7971=EDGE_CURVE ( 'NONE', #1691, #13383, #3434, .T. ) ;
#7983=FACE_OUTER_BOUND ( 'NONE', #9737, .T. ) ;
#7998=DIRECTION ( 'NONE',  ( 0.000000000000000000, 1.000000000000000000, -0.000000000000000000 ) ) ;
#8002=CARTESIAN_POINT ( 'NONE',  ( 118.0000000000000284, 19.25070940071370273, -13.14990448602693007 ) ) ;
#8005=DIRECTION ( 'NONE',  ( -1.000000000000000000, -1.156482317317870492E-16, 0.000000000000000000 ) ) ;
#8014=DIRECTION ( 'NONE',  ( 0.000000000000000000, 0.000000000000000000, 1.000000000000000000 ) ) ;
#8016=DIRECTION ( 'NONE',  ( 0.000000000000000000, -0.000000000000000000, 1.000000000000000000 ) ) ;
#8018=ORIENTED_EDGE ( 'NONE', *, *, #1457, .T. ) ;
#8021=CARTESIAN_POINT ( 'NONE',  ( 51.75774672102440377, 23.25070940071368852, -33.00000000000012790 ) ) ;
#8024=DIRECTION ( 'NONE',  ( 1.156482317317870492E-16, -1.000000000000000000, 0.000000000000000000 ) ) ;
#8025=CARTESIAN_POINT ( 'NONE',  ( 98.40734512546775647, 21.75070940071359615, -33.00000000000012790 ) ) ;
#8027=CARTESIAN_POINT ( 'NONE',  ( 25.81270058232203013, 21.75070940071309167, 139.1143251403882459 ) ) ;
#8028=AXIS2_PLACEMENT_3D ( 'NONE', #12623, #10544, #4920 ) ;
#8033=FACE_OUTER_BOUND ( 'NONE', #6069, .T. ) ;
#8041=EDGE_CURVE ( 'NONE', #12295, #13132, #9521, .T. ) ;
#8049=CARTESIAN_POINT ( 'NONE',  ( 109.8334623555409735, 21.75070940071366365, -13.14990448602693007 ) ) ;
#8058=( NAMED_UNIT ( * ) PLANE_ANGLE_UNIT ( ) SI_UNIT ( $, .RADIAN. ) );
#8066=DIRECTION ( 'NONE',  ( -0.000000000000000000, -0.000000000000000000, -1.000000000000000000 ) ) ;
#8077=EDGE_CURVE ( 'NONE', #5759, #6007, #11964, .T. ) ;
#8078=VERTEX_POINT ( 'NONE', #14213 ) ;
#8080=CARTESIAN_POINT ( 'NONE',  ( 40.33162949095117966, 21.75070940071319114, -33.00000000000012790 ) ) ;
#8083=LINE ( 'NONE', #11450, #8162 ) ;
#8089=ORIENTED_EDGE ( 'NONE', *, *, #1721, .F. ) ;
#8095=DIRECTION ( 'NONE',  ( 1.000000000000000000, 0.000000000000000000, 0.000000000000000000 ) ) ;
#8103=FACE_OUTER_BOUND ( 'NONE', #3582, .T. ) ;
#8107=DIRECTION ( 'NONE',  ( -1.000000000000000000, 0.000000000000000000, 0.000000000000000000 ) ) ;
#8109=AXIS2_PLACEMENT_3D ( 'NONE', #6618, #11166, #13547 ) ;
#8110=CARTESIAN_POINT ( 'NONE',  ( 18.00000000000001066, 23.25070940071368497, 33.00000000000012790 ) ) ;
#8117=ORIENTED_EDGE ( 'NONE', *, *, #10001, .F. ) ;
#8120=AXIS2_PLACEMENT_3D ( 'NONE', #11310, #925, #5486 ) ;
#8126=EDGE_CURVE ( 'NONE', #14644, #9571, #3733, .T. ) ;
#8128=AXIS2_PLACEMENT_3D ( 'NONE', #5335, #5567, #2869 ) ;
#8130=LINE ( 'NONE', #14976, #7551 ) ;
#8131=ORIENTED_EDGE ( 'NONE', *, *, #10022, .F. ) ;
#8135=EDGE_LOOP ( 'NONE', ( #6993, #8840, #8980, #1848 ) ) ;
#8136=CARTESIAN_POINT ( 'NONE',  ( 0.000000000000000000, 21.75070940071369918, 139.1143251403882459 ) ) ;
#8137=CARTESIAN_POINT ( 'NONE',  ( 103.2469880950108063, 21.75070940071363168, 139.1143251403882459 ) ) ;
#8138=VECTOR ( 'NONE', #6888, 1000.000000000000000 ) ;
#8144=CIRCLE ( 'NONE', #1510, 4.000000000000003553 ) ;
#8146=EDGE_CURVE ( 'NONE', #6460, #9928, #14434, .T. ) ;
#8149=VECTOR ( 'NONE', #11122, 1000.000000000000000 ) ;
#8150=EDGE_LOOP ( 'NONE', ( #460, #2090, #576, #1672 ) ) ;
#8151=AXIS2_PLACEMENT_3D ( 'NONE', #992, #9317, #7859 ) ;
#8158=CARTESIAN_POINT ( 'NONE',  ( -2.688903428702175252E-15, 23.25070940071368142, -33.00000000000012790 ) ) ;
#8162=VECTOR ( 'NONE', #15090, 1000.000000000000000 ) ;
#8163=DIRECTION ( 'NONE',  ( -0.000000000000000000, -0.000000000000000000, -1.000000000000000000 ) ) ;
#8175=VECTOR ( 'NONE', #11407, 1000.000000000000000 ) ;
#8184=VERTEX_POINT ( 'NONE', #5189 ) ;
#8188=VECTOR ( 'NONE', #757, 1000.000000000000000 ) ;
#8190=LINE ( 'NONE', #12892, #2448 ) ;
#8194=EDGE_CURVE ( 'NONE', #4644, #15071, #14576, .T. ) ;
#8197=LINE ( 'NONE', #7031, #7370 ) ;
#8198=ORIENTED_EDGE ( 'NONE', *, *, #8772, .F. ) ;
#8200=FACE_OUTER_BOUND ( 'NONE', #10743, .T. ) ;
#8208=ADVANCED_FACE ( 'NONE', ( #3884 ), #491, .F. ) ;
#8216=ADVANCED_FACE ( 'NONE', ( #8033 ), #5653, .T. ) ;
#8234=VERTEX_POINT ( 'NONE', #2099 ) ;
#8235=DIRECTION ( 'NONE',  ( -0.000000000000000000, -0.000000000000000000, -1.000000000000000000 ) ) ;
#8236=VERTEX_POINT ( 'NONE', #4326 ) ;
#8241=LINE ( 'NONE', #8158, #2119 ) ;
#8242=DIRECTION ( 'NONE',  ( 0.000000000000000000, -0.000000000000000000, -1.000000000000000000 ) ) ;
#8250=CARTESIAN_POINT ( 'NONE',  ( 114.0000000000000284, 19.25070940071369563, 13.14990448602693007 ) ) ;
#8251=ORIENTED_EDGE ( 'NONE', *, *, #5886, .T. ) ;
#8254=DIRECTION ( 'NONE',  ( -1.734723475976807292E-15, 1.000000000000000000, 0.000000000000000000 ) ) ;
#8262=CARTESIAN_POINT ( 'NONE',  ( 118.0000000000000284, 19.25070940071370273, 33.00000000000012790 ) ) ;
#8263=ORIENTED_EDGE ( 'NONE', *, *, #3559, .T. ) ;
#8267=FACE_OUTER_BOUND ( 'NONE', #5384, .T. ) ;
#8270=CARTESIAN_POINT ( 'NONE',  ( 58.00000000000000711, 10.75070940071368852, -33.00000000000012790 ) ) ;
#8271=ORIENTED_EDGE ( 'NONE', *, *, #14983, .F. ) ;
#8273=LINE ( 'NONE', #14349, #13756 ) ;
#8279=LINE ( 'NONE', #4517, #7543 ) ;
#8280=CARTESIAN_POINT ( 'NONE',  ( 104.0000000000000426, 11.25070940071369563, 33.00000000000012790 ) ) ;
#8283=DIRECTION ( 'NONE',  ( 0.000000000000000000, 0.000000000000000000, 1.000000000000000000 ) ) ;
#8288=ORIENTED_EDGE ( 'NONE', *, *, #10463, .T. ) ;
#8289=CARTESIAN_POINT ( 'NONE',  ( 0.000000000000000000, 21.75070940071356418, 33.00000000000012790 ) ) ;
#8310=ORIENTED_EDGE ( 'NONE', *, *, #6594, .T. ) ;
#8312=EDGE_LOOP ( 'NONE', ( #2813, #6217, #10221, #4279 ) ) ;
#8318=ORIENTED_EDGE ( 'NONE', *, *, #1519, .T. ) ;
#8320=VECTOR ( 'NONE', #5560, 1000.000000000000000 ) ;
#8323=ORIENTED_EDGE ( 'NONE', *, *, #5626, .T. ) ;
#8325=DIRECTION ( 'NONE',  ( 1.000000000000000000, 0.000000000000000000, 0.000000000000000000 ) ) ;
#8326=FACE_OUTER_BOUND ( 'NONE', #14902, .T. ) ;
#8331=ORIENTED_EDGE ( 'NONE', *, *, #9993, .F. ) ;
#8346=LINE ( 'NONE', #8561, #1551 ) ;
#8351=CARTESIAN_POINT ( 'NONE',  ( 25.81270058232203013, 21.75070940071309167, 33.00000000000012790 ) ) ;
#8353=DIRECTION ( 'NONE',  ( 1.156482317317870492E-16, -1.000000000000000000, 0.000000000000000000 ) ) ;
#8355=DIRECTION ( 'NONE',  ( -0.000000000000000000, -0.000000000000000000, -1.000000000000000000 ) ) ;
#8359=VECTOR ( 'NONE', #4460, 1000.000000000000000 ) ;
#8365=ORIENTED_EDGE ( 'NONE', *, *, #5794, .F. ) ;
#8367=ORIENTED_EDGE ( 'NONE', *, *, #13911, .T. ) ;
#8368=CARTESIAN_POINT ( 'NONE',  ( 35.49198652140812982, 0.000000000000000000, 33.00000000000012790 ) ) ;
#8372=CARTESIAN_POINT ( 'NONE',  ( 104.9938193859979236, 23.25070940071369208, 33.00000000000012790 ) ) ;
#8375=MECHANICAL_DESIGN_GEOMETRIC_PRESENTATION_REPRESENTATION('',(#13046),#8842);
#8380=CARTESIAN_POINT ( 'NONE',  ( 18.00000000000001066, 23.25070940071368497, 139.1143251403882459 ) ) ;
#8390=EDGE_CURVE ( 'NONE', #9917, #4237, #8197, .T. ) ;
#8391=CARTESIAN_POINT ( 'NONE',  ( 25.81270058232203013, 23.25070940071368852, -33.00000000000012790 ) ) ;
#8392=DIRECTION ( 'NONE',  ( -0.000000000000000000, 0.000000000000000000, -1.000000000000000000 ) ) ;
#8394=LINE ( 'NONE', #13087, #2993 ) ;
#8397=EDGE_CURVE ( 'NONE', #14241, #77, #8273, .T. ) ;
#8402=VERTEX_POINT ( 'NONE', #8351 ) ;
#8406=VECTOR ( 'NONE', #1146, 1000.000000000000000 ) ;
#8408=LINE ( 'NONE', #3477, #2847 ) ;
#8410=AXIS2_PLACEMENT_3D ( 'NONE', #14430, #9300, #9455 ) ;
#8418=DIRECTION ( 'NONE',  ( -1.000000000000000000, 0.000000000000000000, 0.000000000000000000 ) ) ;
#8419=CARTESIAN_POINT ( 'NONE',  ( 114.0000000000000284, 19.25070940071369563, 139.1143251403882459 ) ) ;
#8426=PLANE ( 'NONE',  #42 ) ;
#8428=ADVANCED_FACE ( 'NONE', ( #9427 ), #11878, .T. ) ;
#8429=EDGE_LOOP ( 'NONE', ( #12537, #2598, #14078, #4683 ) ) ;
#8431=CARTESIAN_POINT ( 'NONE',  ( 93.56770215592470663, 21.75070940071356418, 139.1143251403882459 ) ) ;
#8437=EDGE_CURVE ( 'NONE', #13017, #14235, #13040, .T. ) ;
#8440=LINE ( 'NONE', #4890, #10769 ) ;
#8445=AXIS2_PLACEMENT_3D ( 'NONE', #3819, #10915, #8591 ) ;
#8447=VECTOR ( 'NONE', #13141, 1000.000000000000000 ) ;
#8457=DIRECTION ( 'NONE',  ( 0.000000000000000000, 1.000000000000000000, -0.000000000000000000 ) ) ;
#8464=ORIENTED_EDGE ( 'NONE', *, *, #5917, .T. ) ;
#8465=DIRECTION ( 'NONE',  ( 0.000000000000000000, -0.000000000000000000, 1.000000000000000000 ) ) ;
#8468=VERTEX_POINT ( 'NONE', #12108 ) ;
#8474=CARTESIAN_POINT ( 'NONE',  ( 0.000000000000000000, 21.75070940071315562, -33.00000000000012790 ) ) ;
#8479=DIRECTION ( 'NONE',  ( 1.000000000000000000, 0.000000000000000000, 0.000000000000000000 ) ) ;
#8487=EDGE_CURVE ( 'NONE', #2597, #1844, #14420, .T. ) ;
#8488=ORIENTED_EDGE ( 'NONE', *, *, #12870, .F. ) ;
#8491=DIRECTION ( 'NONE',  ( 0.000000000000000000, 1.000000000000000000, -0.000000000000000000 ) ) ;
#8494=CARTESIAN_POINT ( 'NONE',  ( 114.6731053250840233, 23.25070940071369563, 33.00000000000012790 ) ) ;
#8511=APPLICATION_CONTEXT ( 'automotive_design' ) ;
#8517=LINE ( 'NONE', #2667, #13198 ) ;
#8522=FACE_OUTER_BOUND ( 'NONE', #14574, .T. ) ;
#8528=ADVANCED_FACE ( 'NONE', ( #1707 ), #7635, .T. ) ;
#8529=LINE ( 'NONE', #8380, #11218 ) ;
#8530=EDGE_CURVE ( 'NONE', #8969, #3666, #2794, .T. ) ;
#8536=VERTEX_POINT ( 'NONE', #13397 ) ;
#8550=VECTOR ( 'NONE', #12389, 1000.000000000000000 ) ;
#8552=DIRECTION ( 'NONE',  ( -1.000000000000000000, -1.734723475976807292E-15, 0.000000000000000000 ) ) ;
#8560=LINE ( 'NONE', #398, #7120 ) ;
#8561=CARTESIAN_POINT ( 'NONE',  ( 104.9938193859979236, 0.000000000000000000, -33.00000000000012790 ) ) ;
#8563=CARTESIAN_POINT ( 'NONE',  ( 27.55953187330915810, 0.000000000000000000, 139.1143251403882459 ) ) ;
#8565=CARTESIAN_POINT ( 'NONE',  ( 42.07846078193830408, 23.25070940071368852, 139.1143251403882459 ) ) ;
#8567=DIRECTION ( 'NONE',  ( 0.000000000000000000, 0.000000000000000000, 1.000000000000000000 ) ) ;
#8569=ADVANCED_FACE ( 'NONE', ( #9011 ), #14783, .F. ) ;
#8572=EDGE_CURVE ( 'NONE', #14721, #5437, #847, .T. ) ;
#8575=ADVANCED_FACE ( 'NONE', ( #3164 ), #6852, .T. ) ;
#8587=AXIS2_PLACEMENT_3D ( 'NONE', #12480, #7946, #2165 ) ;
#8591=DIRECTION ( 'NONE',  ( 0.000000000000000000, 0.000000000000000000, 1.000000000000000000 ) ) ;
#8592=CARTESIAN_POINT ( 'NONE',  ( 118.0000000000000284, 23.25070940071369563, -33.00000000000012790 ) ) ;
#8595=ORIENTED_EDGE ( 'NONE', *, *, #7333, .T. ) ;
#8597=FACE_OUTER_BOUND ( 'NONE', #10153, .T. ) ;
#8599=CARTESIAN_POINT ( 'NONE',  ( 114.0000000000000284, 15.25070940071369563, 13.14990448602693007 ) ) ;
#8604=FACE_OUTER_BOUND ( 'NONE', #1289, .T. ) ;
#8613=LINE ( 'NONE', #12083, #7953 ) ;
#8623=EDGE_CURVE ( 'NONE', #3925, #13020, #2084, .T. ) ;
#8639=VECTOR ( 'NONE', #620, 1000.000000000000000 ) ;
#8641=VECTOR ( 'NONE', #2611, 1000.000000000000000 ) ;
#8644=CARTESIAN_POINT ( 'NONE',  ( 108.0866310645538562, 21.75070940071366365, 139.1143251403882459 ) ) ;
#8645=LINE ( 'NONE', #11755, #10366 ) ;
#8646=EDGE_CURVE ( 'NONE', #1117, #2307, #6775, .T. ) ;
#8653=LINE ( 'NONE', #7575, #10117 ) ;
#8655=VECTOR ( 'NONE', #7792, 1000.000000000000000 ) ;
#8663=AXIS2_PLACEMENT_3D ( 'NONE', #7359, #9968, #5195 ) ;
#8673=ORIENTED_EDGE ( 'NONE', *, *, #8934, .T. ) ;
#8684=DIRECTION ( 'NONE',  ( 1.156482317317870492E-16, -1.000000000000000000, 0.000000000000000000 ) ) ;
#8694=LINE ( 'NONE', #7397, #14311 ) ;
#8707=ORIENTED_EDGE ( 'NONE', *, *, #1222, .F. ) ;
#8708=FACE_OUTER_BOUND ( 'NONE', #13358, .T. ) ;
#8721=DIRECTION ( 'NONE',  ( 0.000000000000000000, -0.000000000000000000, 1.000000000000000000 ) ) ;
#8722=ORIENTED_EDGE ( 'NONE', *, *, #13610, .T. ) ;
#8728=VECTOR ( 'NONE', #5729, 1000.000000000000000 ) ;
#8736=VERTEX_POINT ( 'NONE', #9846 ) ;
#8755=FACE_OUTER_BOUND ( 'NONE', #8429, .T. ) ;
#8771=VECTOR ( 'NONE', #13855, 1000.000000000000000 ) ;
#8772=EDGE_CURVE ( 'NONE', #2535, #7467, #7831, .T. ) ;
#8775=ORIENTED_EDGE ( 'NONE', *, *, #9435, .F. ) ;
#8777=CARTESIAN_POINT ( 'NONE',  ( 118.0000000000000284, 23.25070940071369563, -13.14990448602692474 ) ) ;
#8788=AXIS2_PLACEMENT_3D ( 'NONE', #7462, #12149, #10995 ) ;
#8795=VECTOR ( 'NONE', #14997, 1000.000000000000000 ) ;
#8798=VERTEX_POINT ( 'NONE', #812 ) ;
#8801=ORIENTED_EDGE ( 'NONE', *, *, #14768, .T. ) ;
#8803=ORIENTED_EDGE ( 'NONE', *, *, #1872, .F. ) ;
#8814=ORIENTED_EDGE ( 'NONE', *, *, #6928, .T. ) ;
#8828=VECTOR ( 'NONE', #9879, 1000.000000000000000 ) ;
#8833=ORIENTED_EDGE ( 'NONE', *, *, #4799, .T. ) ;
#8836=EDGE_LOOP ( 'NONE', ( #2096, #4284, #14940, #12346 ) ) ;
#8837=ORIENTED_EDGE ( 'NONE', *, *, #3399, .T. ) ;
#8840=ORIENTED_EDGE ( 'NONE', *, *, #3608, .T. ) ;
#8842=( GEOMETRIC_REPRESENTATION_CONTEXT ( 3 ) GLOBAL_UNCERTAINTY_ASSIGNED_CONTEXT ( ( #5045 ) ) GLOBAL_UNIT_ASSIGNED_CONTEXT ( ( #13903, #8058, #2955 ) ) REPRESENTATION_CONTEXT ( 'NONE', 'WORKASPACE' ) );
#8844=DIRECTION ( 'NONE',  ( 0.000000000000000000, 0.000000000000000000, 1.000000000000000000 ) ) ;
#8850=DIRECTION ( 'NONE',  ( 1.000000000000000000, 0.000000000000000000, -0.000000000000000000 ) ) ;
#8854=LINE ( 'NONE', #14559, #4910 ) ;
#8855=ORIENTED_EDGE ( 'NONE', *, *, #5121, .F. ) ;
#8858=DIRECTION ( 'NONE',  ( -1.000000000000000000, -8.673617379884035472E-17, 0.000000000000000000 ) ) ;
#8861=DIRECTION ( 'NONE',  ( 8.673617379884035472E-17, -1.000000000000000000, 0.000000000000000000 ) ) ;
#8875=ORIENTED_EDGE ( 'NONE', *, *, #12675, .F. ) ;
#8877=DIRECTION ( 'NONE',  ( 0.000000000000000000, 1.000000000000000000, 0.000000000000000000 ) ) ;
#8881=DIRECTION ( 'NONE',  ( 0.000000000000000000, 0.000000000000000000, 1.000000000000000000 ) ) ;
#8892=CARTESIAN_POINT ( 'NONE',  ( 68.00000000000001421, -2.249290599286293268, 139.1143251403882459 ) ) ;
#8895=CARTESIAN_POINT ( 'NONE',  ( 88.00000000000002842, 9.769962616701380080E-14, -33.00000000000012790 ) ) ;
#8909=ORIENTED_EDGE ( 'NONE', *, *, #15062, .T. ) ;
#8913=DIRECTION ( 'NONE',  ( -0.000000000000000000, -0.000000000000000000, -1.000000000000000000 ) ) ;
#8925=LINE ( 'NONE', #2544, #8641 ) ;
#8934=EDGE_CURVE ( 'NONE', #1117, #11541, #15213, .T. ) ;
#8937=EDGE_CURVE ( 'NONE', #9290, #15116, #10368, .T. ) ;
#8947=MANIFOLD_SOLID_BREP ( 'Fillet12', #5353 ) ;
#8955=VERTEX_POINT ( 'NONE', #10032 ) ;
#8956=PLANE ( 'NONE',  #3224 ) ;
#8958=VERTEX_POINT ( 'NONE', #10108 ) ;
#8965=LINE ( 'NONE', #2197, #8138 ) ;
#8969=VERTEX_POINT ( 'NONE', #4320 ) ;
#8977=DIRECTION ( 'NONE',  ( 0.000000000000000000, -1.000000000000000000, 0.000000000000000000 ) ) ;
#8980=ORIENTED_EDGE ( 'NONE', *, *, #10139, .T. ) ;
#8981=FACE_OUTER_BOUND ( 'NONE', #3001, .T. ) ;
#8985=DIRECTION ( 'NONE',  ( 1.000000000000000000, 8.673617379884035472E-17, 0.000000000000000000 ) ) ;
#8992=VERTEX_POINT ( 'NONE', #628 ) ;
#8994=PLANE ( 'NONE',  #1773 ) ;
#9007=EDGE_LOOP ( 'NONE', ( #389, #2150, #2055, #37 ) ) ;
#9010=VECTOR ( 'NONE', #6060, 1000.000000000000000 ) ;
#9011=FACE_OUTER_BOUND ( 'NONE', #11817, .T. ) ;
#9019=CARTESIAN_POINT ( 'NONE',  ( 95.31453344691183815, 0.000000000000000000, 33.00000000000012790 ) ) ;
#9027=CARTESIAN_POINT ( 'NONE',  ( 0.000000000000000000, 21.75070940071322667, 33.00000000000012790 ) ) ;
#9033=ADVANCED_FACE ( 'NONE', ( #862 ), #1860, .F. ) ;
#9035=CARTESIAN_POINT ( 'NONE',  ( 114.6731053250840233, 0.000000000000000000, -13.14990448602693007 ) ) ;
#9041=DIRECTION ( 'NONE',  ( -1.000000000000000000, -1.156482317317870492E-16, 0.000000000000000000 ) ) ;
#9048=LINE ( 'NONE', #11657, #1254 ) ;
#9050=DIRECTION ( 'NONE',  ( 0.000000000000000000, 1.000000000000000000, -0.000000000000000000 ) ) ;
#9051=DIRECTION ( 'NONE',  ( -0.000000000000000000, -0.000000000000000000, 1.000000000000000000 ) ) ;
#9056=ORIENTED_EDGE ( 'NONE', *, *, #3453, .F. ) ;
#9058=LINE ( 'NONE', #13751, #12697 ) ;
#9076=LINE ( 'NONE', #7700, #320 ) ;
#9096=DIRECTION ( 'NONE',  ( 1.000000000000000000, 0.000000000000000000, 0.000000000000000000 ) ) ;
#9102=DIRECTION ( 'NONE',  ( -1.000000000000000000, -8.673617379884035472E-17, 0.000000000000000000 ) ) ;
#9120=CARTESIAN_POINT ( 'NONE',  ( 114.0000000000000284, 19.25070940071369563, -13.14990448602693007 ) ) ;
#9122=CARTESIAN_POINT ( 'NONE',  ( 109.8334623555409735, 21.75070940071366365, -33.00000000000012790 ) ) ;
#9134=VECTOR ( 'NONE', #8163, 1000.000000000000000 ) ;
#9136=EDGE_CURVE ( 'NONE', #8402, #9446, #9340, .T. ) ;
#9138=AXIS2_PLACEMENT_3D ( 'NONE', #8280, #7969, #15124 ) ;
#9140=CARTESIAN_POINT ( 'NONE',  ( 30.65234355186507997, 0.000000000000000000, -33.00000000000012790 ) ) ;
#9146=AXIS2_PLACEMENT_3D ( 'NONE', #12715, #3476, #8016 ) ;
#9148=VECTOR ( 'NONE', #1379, 1000.000000000000000 ) ;
#9157=CARTESIAN_POINT ( 'NONE',  ( 108.0866310645538562, 23.25070940071369563, 139.1143251403882459 ) ) ;
#9163=AXIS2_PLACEMENT_3D ( 'NONE', #10714, #7247, #13030 ) ;
#9169=DIRECTION ( 'NONE',  ( 0.000000000000000000, 0.000000000000000000, 1.000000000000000000 ) ) ;
#9170=LINE ( 'NONE', #1846, #8359 ) ;
#9181=( LENGTH_UNIT ( ) NAMED_UNIT ( * ) SI_UNIT ( .MILLI., .METRE. ) );
#9185=DIRECTION ( 'NONE',  ( 8.673617379884035472E-17, -1.000000000000000000, 0.000000000000000000 ) ) ;
#9186=VECTOR ( 'NONE', #1733, 1000.000000000000000 ) ;
#9198=VERTEX_POINT ( 'NONE', #14032 ) ;
#9215=CARTESIAN_POINT ( 'NONE',  ( 18.00000000000001066, 15.25070940071368497, -33.00000000000012790 ) ) ;
#9219=DIRECTION ( 'NONE',  ( -0.000000000000000000, -0.000000000000000000, -1.000000000000000000 ) ) ;
#9234=VERTEX_POINT ( 'NONE', #10492 ) ;
#9240=ORIENTED_EDGE ( 'NONE', *, *, #4997, .T. ) ;
#9242=VECTOR ( 'NONE', #12803, 1000.000000000000000 ) ;
#9274=DIRECTION ( 'NONE',  ( 0.000000000000000000, 0.000000000000000000, 1.000000000000000000 ) ) ;
#9275=VECTOR ( 'NONE', #7116, 1000.000000000000000 ) ;
#9280=VECTOR ( 'NONE', #2044, 1000.000000000000000 ) ;
#9284=ADVANCED_FACE ( 'NONE', ( #13400 ), #481, .F. ) ;
#9290=VERTEX_POINT ( 'NONE', #1570 ) ;
#9300=DIRECTION ( 'NONE',  ( -0.000000000000000000, -0.000000000000000000, -1.000000000000000000 ) ) ;
#9317=DIRECTION ( 'NONE',  ( 0.000000000000000000, 1.000000000000000000, 0.000000000000000000 ) ) ;
#9324=ORIENTED_EDGE ( 'NONE', *, *, #14052, .F. ) ;
#9325=CARTESIAN_POINT ( 'NONE',  ( 88.00000000000002842, 9.769962616701380080E-14, 139.1143251403882459 ) ) ;
#9326=AXIS2_PLACEMENT_3D ( 'NONE', #541, #9947, #12170 ) ;
#9340=LINE ( 'NONE', #8027, #13262 ) ;
#9343=CARTESIAN_POINT ( 'NONE',  ( 37.23881781239525424, 0.000000000000000000, 139.1143251403882459 ) ) ;
#9353=DIRECTION ( 'NONE',  ( -0.000000000000000000, -0.000000000000000000, -1.000000000000000000 ) ) ;
#9365=ADVANCED_FACE ( 'NONE', ( #4310 ), #13944, .F. ) ;
#9369=ORIENTED_EDGE ( 'NONE', *, *, #13610, .F. ) ;
#9371=CYLINDRICAL_SURFACE ( 'NONE', #11439, 10.00000000000000178 ) ;
#9372=VECTOR ( 'NONE', #3429, 1000.000000000000000 ) ;
#9377=CARTESIAN_POINT ( 'NONE',  ( 58.00000000000000711, 0.000000000000000000, 139.1143251403882459 ) ) ;
#9380=ORIENTED_EDGE ( 'NONE', *, *, #2415, .F. ) ;
#9381=ORIENTED_EDGE ( 'NONE', *, *, #2820, .F. ) ;
#9382=ADVANCED_FACE ( 'NONE', ( #14860 ), #10098, .F. ) ;
#9383=VECTOR ( 'NONE', #1308, 1000.000000000000000 ) ;
#9402=ORIENTED_EDGE ( 'NONE', *, *, #13911, .F. ) ;
#9422=EDGE_CURVE ( 'NONE', #4285, #844, #13632, .T. ) ;
#9427=FACE_OUTER_BOUND ( 'NONE', #12987, .T. ) ;
#9429=DIRECTION ( 'NONE',  ( 0.000000000000000000, -0.000000000000000000, 1.000000000000000000 ) ) ;
#9432=DIRECTION ( 'NONE',  ( 0.000000000000000000, 1.000000000000000000, -0.000000000000000000 ) ) ;
#9435=EDGE_CURVE ( 'NONE', #8992, #5383, #11782, .T. ) ;
#9446=VERTEX_POINT ( 'NONE', #696 ) ;
#9447=PLANE ( 'NONE',  #10362 ) ;
#9451=DIRECTION ( 'NONE',  ( -0.000000000000000000, -0.000000000000000000, -1.000000000000000000 ) ) ;
#9455=DIRECTION ( 'NONE',  ( -1.000000000000000000, 0.000000000000000000, 0.000000000000000000 ) ) ;
#9458=DIRECTION ( 'NONE',  ( -0.000000000000000000, -0.000000000000000000, -1.000000000000000000 ) ) ;
#9459=ORIENTED_EDGE ( 'NONE', *, *, #12327, .T. ) ;
#9469=CARTESIAN_POINT ( 'NONE',  ( 130.4454129427046496, -1.749290599286305259, -13.14990448602692474 ) ) ;
#9479=CARTESIAN_POINT ( 'NONE',  ( 108.0866310645538562, 21.75070940071366365, 139.1143251403882459 ) ) ;
#9481=PLANE ( 'NONE',  #2265 ) ;
#9492=AXIS2_PLACEMENT_3D ( 'NONE', #6864, #1012, #5802 ) ;
#9508=VECTOR ( 'NONE', #3461, 1000.000000000000000 ) ;
#9511=LINE ( 'NONE', #47, #12997 ) ;
#9518=EDGE_LOOP ( 'NONE', ( #3297, #9459, #14161, #10523 ) ) ;
#9519=EDGE_CURVE ( 'NONE', #1506, #1905, #8408, .T. ) ;
#9521=LINE ( 'NONE', #10818, #10256 ) ;
#9534=VECTOR ( 'NONE', #7294, 1000.000000000000000 ) ;
#9537=CARTESIAN_POINT ( 'NONE',  ( 50.01091543003727224, 23.25070940071368852, 33.00000000000012790 ) ) ;
#9539=VERTEX_POINT ( 'NONE', #10562 ) ;
#9557=EDGE_LOOP ( 'NONE', ( #209, #6915, #12633, #6526 ) ) ;
#9570=EDGE_LOOP ( 'NONE', ( #9381, #6735, #10861, #2201 ) ) ;
#9571=VERTEX_POINT ( 'NONE', #249 ) ;
#9578=DIRECTION ( 'NONE',  ( 0.000000000000000000, -0.000000000000000000, 1.000000000000000000 ) ) ;
#9582=EDGE_CURVE ( 'NONE', #7515, #1460, #9645, .T. ) ;
#9586=DIRECTION ( 'NONE',  ( 1.000000000000000000, 1.156482317317870492E-16, 0.000000000000000000 ) ) ;
#9589=CARTESIAN_POINT ( 'NONE',  ( 40.33162949095117966, 0.000000000000000000, -33.00000000000012790 ) ) ;
#9598=VERTEX_POINT ( 'NONE', #1472 ) ;
#9603=ORIENTED_EDGE ( 'NONE', *, *, #4449, .T. ) ;
#9606=EDGE_CURVE ( 'NONE', #12466, #9700, #12370, .T. ) ;
#9618=LINE ( 'NONE', #14301, #4085 ) ;
#9633=ORIENTED_EDGE ( 'NONE', *, *, #14778, .F. ) ;
#9634=VECTOR ( 'NONE', #14720, 1000.000000000000000 ) ;
#9645=LINE ( 'NONE', #3398, #5313 ) ;
#9646=ORIENTED_EDGE ( 'NONE', *, *, #10279, .T. ) ;
#9654=CARTESIAN_POINT ( 'NONE',  ( 100.1541764164548880, 23.25070940071369208, -33.00000000000012790 ) ) ;
#9661=EDGE_CURVE ( 'NONE', #11505, #1679, #4274, .T. ) ;
#9676=EDGE_CURVE ( 'NONE', #1446, #4646, #813, .T. ) ;
#9683=EDGE_LOOP ( 'NONE', ( #2294, #12691, #11252, #7574, #11981, #2950, #10326, #4363 ) ) ;
#9684=DIRECTION ( 'NONE',  ( -0.000000000000000000, -0.000000000000000000, 1.000000000000000000 ) ) ;
#9690=FACE_OUTER_BOUND ( 'NONE', #6350, .T. ) ;
#9691=ORIENTED_EDGE ( 'NONE', *, *, #2750, .T. ) ;
#9696=VECTOR ( 'NONE', #11681, 1000.000000000000000 ) ;
#9699=ORIENTED_EDGE ( 'NONE', *, *, #3344, .F. ) ;
#9700=VERTEX_POINT ( 'NONE', #659 ) ;
#9701=DIRECTION ( 'NONE',  ( 0.000000000000000000, 1.000000000000000000, 0.000000000000000000 ) ) ;
#9705=ORIENTED_EDGE ( 'NONE', *, *, #6853, .T. ) ;
#9717=ORIENTED_EDGE ( 'NONE', *, *, #335, .F. ) ;
#9719=ADVANCED_FACE ( 'NONE', ( #5443 ), #10138, .T. ) ;
#9737=EDGE_LOOP ( 'NONE', ( #2424, #8323, #3085, #1537 ) ) ;
#9738=LINE ( 'NONE', #7945, #10129 ) ;
#9752=ORIENTED_EDGE ( 'NONE', *, *, #7758, .T. ) ;
#9753=FACE_OUTER_BOUND ( 'NONE', #14255, .T. ) ;
#9755=CARTESIAN_POINT ( 'NONE',  ( 58.00000000000000711, 10.75070940071368852, 139.1143251403882459 ) ) ;
#9756=EDGE_CURVE ( 'NONE', #13017, #11141, #5600, .T. ) ;
#9762=FACE_OUTER_BOUND ( 'NONE', #11927, .T. ) ;
#9765=ORIENTED_EDGE ( 'NONE', *, *, #3328, .T. ) ;
#9773=ADVANCED_FACE ( 'NONE', ( #7983 ), #9371, .T. ) ;
#9796=ADVANCED_FACE ( 'NONE', ( #2124 ), #2210, .F. ) ;
#9799=LINE ( 'NONE', #537, #1121 ) ;
#9802=VECTOR ( 'NONE', #257, 1000.000000000000000 ) ;
#9805=LINE ( 'NONE', #2635, #3912 ) ;
#9809=EDGE_CURVE ( 'NONE', #3269, #10461, #12763, .T. ) ;
#9827=ORIENTED_EDGE ( 'NONE', *, *, #10832, .T. ) ;
#9831=VECTOR ( 'NONE', #5557, 1000.000000000000000 ) ;
#9834=PLANE ( 'NONE',  #2408 ) ;
#9835=EDGE_CURVE ( 'NONE', #13383, #1549, #9058, .T. ) ;
#9839=AXIS2_PLACEMENT_3D ( 'NONE', #14643, #13569, #7501 ) ;
#9845=ORIENTED_EDGE ( 'NONE', *, *, #525, .F. ) ;
#9846=CARTESIAN_POINT ( 'NONE',  ( 108.0866310645538562, 23.25070940071369563, -33.00000000000012790 ) ) ;
#9848=CARTESIAN_POINT ( 'NONE',  ( -2.016677571526633510E-15, 23.25070940071368497, 139.1143251403882459 ) ) ;
#9851=VECTOR ( 'NONE', #8858, 1000.000000000000000 ) ;
#9855=CARTESIAN_POINT ( 'NONE',  ( 62.00000000000001421, -2.249290599286310588, 33.00000000000012790 ) ) ;
#9858=PRODUCT_DEFINITION ( 'UNKNOWN', '', #15181, #5987 ) ;
#9859=CARTESIAN_POINT ( 'NONE',  ( 100.1541764164548880, 23.25070940071369208, 139.1143251403882459 ) ) ;
#9861=LINE ( 'NONE', #14685, #14694 ) ;
#9863=EDGE_LOOP ( 'NONE', ( #14305, #3840, #3648, #11221 ) ) ;
#9864=ORIENTED_EDGE ( 'NONE', *, *, #3568, .T. ) ;
#9868=PLANE ( 'NONE',  #3874 ) ;
#9875=LINE ( 'NONE', #14704, #10812 ) ;
#9878=AXIS2_PLACEMENT_3D ( 'NONE', #1091, #8024, #7175 ) ;
#9879=DIRECTION ( 'NONE',  ( 0.000000000000000000, 1.000000000000000000, -0.000000000000000000 ) ) ;
#9884=CARTESIAN_POINT ( 'NONE',  ( 112.9262740340969060, 21.75070940071369918, 139.1143251403882459 ) ) ;
#9892=VECTOR ( 'NONE', #12271, 1000.000000000000000 ) ;
#9902=CARTESIAN_POINT ( 'NONE',  ( 56.59738969056744651, 0.000000000000000000, 139.1143251403882459 ) ) ;
#9914=ORIENTED_EDGE ( 'NONE', *, *, #12736, .T. ) ;
#9917=VERTEX_POINT ( 'NONE', #8372 ) ;
#9928=VERTEX_POINT ( 'NONE', #5995 ) ;
#9933=DIRECTION ( 'NONE',  ( 0.000000000000000000, 1.000000000000000000, 0.000000000000000000 ) ) ;
#9934=ORIENTED_EDGE ( 'NONE', *, *, #13734, .F. ) ;
#9947=DIRECTION ( 'NONE',  ( 0.000000000000000000, 0.000000000000000000, 1.000000000000000000 ) ) ;
#9953=ORIENTED_EDGE ( 'NONE', *, *, #12230, .T. ) ;
#9956=EDGE_CURVE ( 'NONE', #11167, #3925, #7282, .T. ) ;
#9967=ORIENTED_EDGE ( 'NONE', *, *, #9676, .T. ) ;
#9968=DIRECTION ( 'NONE',  ( -1.000000000000000000, 0.000000000000000000, 0.000000000000000000 ) ) ;
#9970=LINE ( 'NONE', #6728, #8149 ) ;
#9977=CARTESIAN_POINT ( 'NONE',  ( 109.8334623555409735, 23.25070940071369563, 13.14990448602692474 ) ) ;
#9981=EDGE_CURVE ( 'NONE', #77, #10905, #8517, .T. ) ;
#9983=ORIENTED_EDGE ( 'NONE', *, *, #13106, .T. ) ;
#9987=DIRECTION ( 'NONE',  ( 1.000000000000000000, 8.673617379884035472E-17, 0.000000000000000000 ) ) ;
#9990=CARTESIAN_POINT ( 'NONE',  ( 100.1541764164548880, 21.75070940071359615, 33.00000000000012790 ) ) ;
#9992=AXIS2_PLACEMENT_3D ( 'NONE', #1893, #11427, #6513 ) ;
#9993=EDGE_CURVE ( 'NONE', #7396, #2597, #12131, .T. ) ;
#10001=EDGE_CURVE ( 'NONE', #72, #5415, #6500, .T. ) ;
#10007=CARTESIAN_POINT ( 'NONE',  ( 104.9938193859979236, 21.75070940071363168, 139.1143251403882459 ) ) ;
#10012=ADVANCED_FACE ( 'NONE', ( #5348 ), #13653, .T. ) ;
#10022=EDGE_CURVE ( 'NONE', #3269, #12669, #10119, .T. ) ;
#10025=CARTESIAN_POINT ( 'NONE',  ( -2.016677571526633510E-15, 23.25070940071368497, 139.1143251403882459 ) ) ;
#10032=CARTESIAN_POINT ( 'NONE',  ( 112.9262740340969060, 21.75070940071369918, 13.14990448602693007 ) ) ;
#10037=VECTOR ( 'NONE', #273, 1000.000000000000000 ) ;
#10039=DIRECTION ( 'NONE',  ( -0.000000000000000000, -0.000000000000000000, -1.000000000000000000 ) ) ;
#10041=CARTESIAN_POINT ( 'NONE',  ( -1.243300532054838308E-15, 10.75070940071368142, 139.1143251403882459 ) ) ;
#10042=CARTESIAN_POINT ( 'NONE',  ( 68.00000000000000000, 2.750709400713692965, -33.00000000000012790 ) ) ;
#10049=AXIS2_PLACEMENT_3D ( 'NONE', #3987, #7234, #8684 ) ;
#10052=ORIENTED_EDGE ( 'NONE', *, *, #6882, .T. ) ;
#10059=ORIENTED_EDGE ( 'NONE', *, *, #7721, .F. ) ;
#10061=CARTESIAN_POINT ( 'NONE',  ( 98.40734512546775647, 21.75070940071359615, 139.1143251403882459 ) ) ;
#10064=ORIENTED_EDGE ( 'NONE', *, *, #7971, .F. ) ;
#10066=VERTEX_POINT ( 'NONE', #6356 ) ;
#10072=LINE ( 'NONE', #6675, #2042 ) ;
#10074=VERTEX_POINT ( 'NONE', #12352 ) ;
#10077=ORIENTED_EDGE ( 'NONE', *, *, #12339, .F. ) ;
#10093=ORIENTED_EDGE ( 'NONE', *, *, #7446, .T. ) ;
#10098=PLANE ( 'NONE',  #1938 ) ;
#10102=EDGE_LOOP ( 'NONE', ( #11093, #2778, #391, #9633 ) ) ;
#10103=CARTESIAN_POINT ( 'NONE',  ( 105.5545870572953930, 23.25070940071369563, -13.14990448602692474 ) ) ;
#10107=LINE ( 'NONE', #6866, #6142 ) ;
#10108=CARTESIAN_POINT ( 'NONE',  ( 109.8334623555409735, 23.25070940071369563, -13.14990448602692474 ) ) ;
#10114=CARTESIAN_POINT ( 'NONE',  ( -2.688903428702175252E-15, 23.25070940071368142, -33.00000000000012790 ) ) ;
#10117=VECTOR ( 'NONE', #7655, 1000.000000000000000 ) ;
#10119=LINE ( 'NONE', #4259, #14903 ) ;
#10129=VECTOR ( 'NONE', #9096, 1000.000000000000000 ) ;
#10136=ORIENTED_EDGE ( 'NONE', *, *, #10488, .F. ) ;
#10138=PLANE ( 'NONE',  #402 ) ;
#10139=EDGE_CURVE ( 'NONE', #5383, #2542, #10197, .T. ) ;
#10153=EDGE_LOOP ( 'NONE', ( #5952, #9953, #10899, #11422 ) ) ;
#10156=ORIENTED_EDGE ( 'NONE', *, *, #1364, .T. ) ;
#10174=FACE_OUTER_BOUND ( 'NONE', #10525, .T. ) ;
#10175=CARTESIAN_POINT ( 'NONE',  ( 50.01091543003727224, 23.25070940071368852, 139.1143251403882459 ) ) ;
#10182=ORIENTED_EDGE ( 'NONE', *, *, #12197, .F. ) ;
#10183=DIRECTION ( 'NONE',  ( -0.000000000000000000, -0.000000000000000000, -1.000000000000000000 ) ) ;
#10197=LINE ( 'NONE', #4414, #6791 ) ;
#10201=LINE ( 'NONE', #6732, #3948 ) ;
#10210=EDGE_LOOP ( 'NONE', ( #10615, #2932, #5011, #7594 ) ) ;
#10214=LINE ( 'NONE', #3131, #3539 ) ;
#10216=EDGE_LOOP ( 'NONE', ( #8117, #1559, #10828, #14134, #1445, #11530, #13797, #3364, #2685, #5002, #3221, #6478, #7184 ) ) ;
#10221=ORIENTED_EDGE ( 'NONE', *, *, #12225, .F. ) ;
#10226=ORIENTED_EDGE ( 'NONE', *, *, #2123, .F. ) ;
#10235=DIRECTION ( 'NONE',  ( -0.000000000000000000, -0.000000000000000000, -1.000000000000000000 ) ) ;
#10242=EDGE_LOOP ( 'NONE', ( #10469, #7028, #9967, #1674 ) ) ;
#10247=EDGE_CURVE ( 'NONE', #72, #4346, #13430, .T. ) ;
#10252=( NAMED_UNIT ( * ) SI_UNIT ( $, .STERADIAN. ) SOLID_ANGLE_UNIT ( ) );
#10253=LINE ( 'NONE', #1932, #15186 ) ;
#10256=VECTOR ( 'NONE', #1352, 1000.000000000000000 ) ;
#10267=ORIENTED_EDGE ( 'NONE', *, *, #7083, .T. ) ;
#10275=ORIENTED_EDGE ( 'NONE', *, *, #14302, .T. ) ;
#10278=ADVANCED_FACE ( 'NONE', ( #3341 ), #12744, .F. ) ;
#10279=EDGE_CURVE ( 'NONE', #11241, #13684, #6881, .T. ) ;
#10281=VECTOR ( 'NONE', #7314, 1000.000000000000000 ) ;
#10286=DIRECTION ( 'NONE',  ( -1.000000000000000000, -8.673617379884035472E-17, 0.000000000000000000 ) ) ;
#10287=LINE ( 'NONE', #3278, #7801 ) ;
#10291=CARTESIAN_POINT ( 'NONE',  ( 109.8334623555409735, 23.25070940071369563, -33.00000000000012790 ) ) ;
#10307=LINE ( 'NONE', #13918, #2766 ) ;
#10317=CARTESIAN_POINT ( 'NONE',  ( 25.81270058232203013, 23.25070940071368852, 33.00000000000012790 ) ) ;
#10326=ORIENTED_EDGE ( 'NONE', *, *, #7259, .T. ) ;
#10331=DIRECTION ( 'NONE',  ( -1.000000000000000000, 0.000000000000000000, 0.000000000000000000 ) ) ;
#10333=EDGE_CURVE ( 'NONE', #5415, #10867, #6202, .T. ) ;
#10336=DIRECTION ( 'NONE',  ( 1.000000000000000000, 0.000000000000000000, 0.000000000000000000 ) ) ;
#10345=DIRECTION ( 'NONE',  ( -1.000000000000000000, 0.000000000000000000, 0.000000000000000000 ) ) ;
#10362=AXIS2_PLACEMENT_3D ( 'NONE', #12988, #2436, #11815 ) ;
#10366=VECTOR ( 'NONE', #13344, 1000.000000000000000 ) ;
#10368=LINE ( 'NONE', #9140, #11062 ) ;
#10373=ORIENTED_EDGE ( 'NONE', *, *, #7912, .F. ) ;
#10374=AXIS2_PLACEMENT_3D ( 'NONE', #7035, #12970, #4648 ) ;
#10381=ORIENTED_EDGE ( 'NONE', *, *, #14052, .T. ) ;
#10389=ORIENTED_EDGE ( 'NONE', *, *, #12736, .F. ) ;
#10390=VECTOR ( 'NONE', #1398, 1000.000000000000000 ) ;
#10393=CIRCLE ( 'NONE', #4235, 9.999999999999994671 ) ;
#10398=VECTOR ( 'NONE', #9432, 1000.000000000000000 ) ;
#10403=AXIS2_PLACEMENT_3D ( 'NONE', #9377, #14072, #4761 ) ;
#10417=CARTESIAN_POINT ( 'NONE',  ( 0.000000000000000000, 21.75070940071366365, 13.14990448602693007 ) ) ;
#10418=VECTOR ( 'NONE', #1956, 1000.000000000000000 ) ;
#10429=LINE ( 'NONE', #12578, #11856 ) ;
#10435=CARTESIAN_POINT ( 'NONE',  ( -2.016677571526633510E-15, 23.25070940071368497, 33.00000000000012790 ) ) ;
#10438=ORIENTED_EDGE ( 'NONE', *, *, #6532, .F. ) ;
#10442=DIRECTION ( 'NONE',  ( 0.000000000000000000, 1.000000000000000000, -0.000000000000000000 ) ) ;
#10446=EDGE_CURVE ( 'NONE', #13020, #7467, #41, .T. ) ;
#10447=DIRECTION ( 'NONE',  ( 8.673617379884035472E-17, -1.000000000000000000, 0.000000000000000000 ) ) ;
#10448=CARTESIAN_POINT ( 'NONE',  ( 108.0866310645538562, 23.25070940071369563, -13.14990448602692474 ) ) ;
#10454=CARTESIAN_POINT ( 'NONE',  ( 88.00000000000001421, 10.75070940071369208, 33.00000000000012790 ) ) ;
#10461=VERTEX_POINT ( 'NONE', #1414 ) ;
#10463=EDGE_CURVE ( 'NONE', #11541, #13742, #12973, .T. ) ;
#10469=ORIENTED_EDGE ( 'NONE', *, *, #12810, .F. ) ;
#10488=EDGE_CURVE ( 'NONE', #8992, #1911, #6338, .T. ) ;
#10490=DIRECTION ( 'NONE',  ( 0.000000000000000000, 1.000000000000000000, -0.000000000000000000 ) ) ;
#10492=CARTESIAN_POINT ( 'NONE',  ( 18.00000000000001066, 15.25070940071368497, 33.00000000000012790 ) ) ;
#10502=LINE ( 'NONE', #13189, #3504 ) ;
#10515=CARTESIAN_POINT ( 'NONE',  ( 95.31453344691183815, 21.75070940071356418, -33.00000000000012790 ) ) ;
#10523=ORIENTED_EDGE ( 'NONE', *, *, #6454, .T. ) ;
#10525=EDGE_LOOP ( 'NONE', ( #6918, #6876, #6891, #1927 ) ) ;
#10544=DIRECTION ( 'NONE',  ( 1.156482317317870492E-16, -1.000000000000000000, 0.000000000000000000 ) ) ;
#10548=LINE ( 'NONE', #11918, #9134 ) ;
#10551=CARTESIAN_POINT ( 'NONE',  ( 58.00000000000000711, -2.249290599286311032, 33.00000000000012790 ) ) ;
#10552=CARTESIAN_POINT ( 'NONE',  ( 109.8334623555409735, 0.000000000000000000, 139.1143251403882459 ) ) ;
#10555=EDGE_LOOP ( 'NONE', ( #13798, #868 ) ) ;
#10556=CARTESIAN_POINT ( 'NONE',  ( 108.0866310645538562, 23.25070940071369563, 139.1143251403882459 ) ) ;
#10560=CARTESIAN_POINT ( 'NONE',  ( 48.00000000000000000, -2.664535259100377906E-14, 139.1143251403882459 ) ) ;
#10562=CARTESIAN_POINT ( 'NONE',  ( 45.17127246049422240, 21.75070940071322667, -33.00000000000012790 ) ) ;
#10564=ORIENTED_EDGE ( 'NONE', *, *, #13841, .T. ) ;
#10571=CARTESIAN_POINT ( 'NONE',  ( 114.6731053250840233, 23.25070940071369563, 13.14990448602692474 ) ) ;
#10580=CARTESIAN_POINT ( 'NONE',  ( 0.000000000000000000, 21.75070940071359615, 139.1143251403882459 ) ) ;
#10605=VECTOR ( 'NONE', #6564, 1000.000000000000000 ) ;
#10615=ORIENTED_EDGE ( 'NONE', *, *, #351, .F. ) ;
#10618=VERTEX_POINT ( 'NONE', #6484 ) ;
#10633=ORIENTED_EDGE ( 'NONE', *, *, #7912, .T. ) ;
#10638=CARTESIAN_POINT ( 'NONE',  ( -2.688903428702175252E-15, 23.25070940071368142, -13.14990448602693007 ) ) ;
#10640=CARTESIAN_POINT ( 'NONE',  ( 46.91810375148135392, 0.000000000000000000, 33.00000000000012790 ) ) ;
#10641=ORIENTED_EDGE ( 'NONE', *, *, #9835, .T. ) ;
#10647=EDGE_CURVE ( 'NONE', #1844, #13613, #855, .T. ) ;
#10655=DIRECTION ( 'NONE',  ( -1.000000000000000000, 0.000000000000000000, 0.000000000000000000 ) ) ;
#10674=ORIENTED_EDGE ( 'NONE', *, *, #5278, .F. ) ;
#10675=CARTESIAN_POINT ( 'NONE',  ( 0.000000000000000000, 15.25070940071369563, -33.00000000000012790 ) ) ;
#10682=DIRECTION ( 'NONE',  ( 1.156482317317870492E-16, -1.000000000000000000, 0.000000000000000000 ) ) ;
#10686=ORIENTED_EDGE ( 'NONE', *, *, #6494, .F. ) ;
#10689=ORIENTED_EDGE ( 'NONE', *, *, #10963, .T. ) ;
#10696=DIRECTION ( 'NONE',  ( 0.000000000000000000, 1.000000000000000000, 0.000000000000000000 ) ) ;
#10702=CARTESIAN_POINT ( 'NONE',  ( -2.688903428702175252E-15, 23.25070940071368142, 33.00000000000012790 ) ) ;
#10706=ORIENTED_EDGE ( 'NONE', *, *, #6533, .F. ) ;
#10714=CARTESIAN_POINT ( 'NONE',  ( 32.39917484285220439, 0.000000000000000000, 139.1143251403882459 ) ) ;
#10718=DIRECTION ( 'NONE',  ( 1.000000000000000000, 0.000000000000000000, 0.000000000000000000 ) ) ;
#10720=LINE ( 'NONE', #12104, #86 ) ;
#10727=DIRECTION ( 'NONE',  ( -1.000000000000000000, 0.000000000000000000, 0.000000000000000000 ) ) ;
#10728=CARTESIAN_POINT ( 'NONE',  ( 103.2469880950108063, 21.75070940071363168, 33.00000000000012790 ) ) ;
#10736=CARTESIAN_POINT ( 'NONE',  ( 96.00000000000002842, 6.750709400713692965, 33.00000000000012790 ) ) ;
#10743=EDGE_LOOP ( 'NONE', ( #6485, #8251, #565, #11814 ) ) ;
#10748=EDGE_CURVE ( 'NONE', #11670, #15071, #10253, .T. ) ;
#10758=FACE_BOUND ( 'NONE', #3456, .T. ) ;
#10769=VECTOR ( 'NONE', #197, 1000.000000000000000 ) ;
#10776=LINE ( 'NONE', #236, #13320 ) ;
#10778=EDGE_CURVE ( 'NONE', #10074, #13054, #4553, .T. ) ;
#10785=FACE_OUTER_BOUND ( 'NONE', #11064, .T. ) ;
#10787=CARTESIAN_POINT ( 'NONE',  ( 48.00000000000000000, -2.249290599286307479, -33.00000000000012790 ) ) ;
#10794=EDGE_CURVE ( 'NONE', #11647, #5697, #14257, .T. ) ;
#10800=DIRECTION ( 'NONE',  ( 0.000000000000000000, 1.000000000000000000, -0.000000000000000000 ) ) ;
#10805=ORIENTED_EDGE ( 'NONE', *, *, #14266, .F. ) ;
#10810=CARTESIAN_POINT ( 'NONE',  ( 114.6731053250840233, 23.25070940071369563, -13.14990448602692474 ) ) ;
#10812=VECTOR ( 'NONE', #13394, 1000.000000000000000 ) ;
#10818=CARTESIAN_POINT ( 'NONE',  ( 100.0000000000000284, 0.000000000000000000, -33.00000000000012790 ) ) ;
#10823=ORIENTED_EDGE ( 'NONE', *, *, #3952, .F. ) ;
#10828=ORIENTED_EDGE ( 'NONE', *, *, #431, .F. ) ;
#10832=EDGE_CURVE ( 'NONE', #14864, #6792, #5881, .T. ) ;
#10859=CYLINDRICAL_SURFACE ( 'NONE', #13232, 4.000000000000003553 ) ;
#10861=ORIENTED_EDGE ( 'NONE', *, *, #10778, .T. ) ;
#10867=VERTEX_POINT ( 'NONE', #4864 ) ;
#10876=CARTESIAN_POINT ( 'NONE',  ( 0.000000000000000000, 21.75070940071369918, 13.14990448602693007 ) ) ;
#10884=ORIENTED_EDGE ( 'NONE', *, *, #11367, .T. ) ;
#10885=CARTESIAN_POINT ( 'NONE',  ( 100.0000000000000284, 0.000000000000000000, 139.1143251403882459 ) ) ;
#10890=VECTOR ( 'NONE', #4536, 1000.000000000000000 ) ;
#10892=CARTESIAN_POINT ( 'NONE',  ( 68.00000000000000000, 2.750709400713692965, 33.00000000000012790 ) ) ;
#10899=ORIENTED_EDGE ( 'NONE', *, *, #10946, .F. ) ;
#10903=ORIENTED_EDGE ( 'NONE', *, *, #7106, .T. ) ;
#10905=VERTEX_POINT ( 'NONE', #14480 ) ;
#10906=VERTEX_POINT ( 'NONE', #13254 ) ;
#10915=DIRECTION ( 'NONE',  ( -1.000000000000000000, 0.000000000000000000, 0.000000000000000000 ) ) ;
#10917=EDGE_LOOP ( 'NONE', ( #13003, #4604, #10931, #10136 ) ) ;
#10921=ORIENTED_EDGE ( 'NONE', *, *, #7904, .T. ) ;
#10931=ORIENTED_EDGE ( 'NONE', *, *, #1721, .T. ) ;
#10934=ADVANCED_FACE ( 'NONE', ( #535 ), #9868, .F. ) ;
#10936=CARTESIAN_POINT ( 'NONE',  ( 42.07846078193830408, 21.75070940071319114, 33.00000000000012790 ) ) ;
#10940=DIRECTION ( 'NONE',  ( -0.000000000000000000, -0.000000000000000000, -1.000000000000000000 ) ) ;
#10946=EDGE_CURVE ( 'NONE', #4644, #2314, #14407, .T. ) ;
#10948=DIRECTION ( 'NONE',  ( -0.000000000000000000, -0.000000000000000000, -1.000000000000000000 ) ) ;
#10949=CARTESIAN_POINT ( 'NONE',  ( 104.9938193859979236, 21.75070940071363168, -33.00000000000012790 ) ) ;
#10960=EDGE_CURVE ( 'NONE', #14235, #5016, #5309, .T. ) ;
#10963=EDGE_CURVE ( 'NONE', #977, #7467, #12165, .T. ) ;
#10966=VECTOR ( 'NONE', #5623, 1000.000000000000000 ) ;
#10970=DIRECTION ( 'NONE',  ( 0.000000000000000000, -1.000000000000000000, 0.000000000000000000 ) ) ;
#10971=FACE_OUTER_BOUND ( 'NONE', #11219, .T. ) ;
#10978=DIRECTION ( 'NONE',  ( -0.000000000000000000, 0.000000000000000000, 1.000000000000000000 ) ) ;
#10995=DIRECTION ( 'NONE',  ( 1.000000000000000000, 8.673617379884035472E-17, 0.000000000000000000 ) ) ;
#10996=CARTESIAN_POINT ( 'NONE',  ( 0.000000000000000000, 15.25070940071369563, 139.1143251403882459 ) ) ;
#11009=VECTOR ( 'NONE', #10718, 1000.000000000000000 ) ;
#11022=DIRECTION ( 'NONE',  ( 1.000000000000000000, 0.000000000000000000, -0.000000000000000000 ) ) ;
#11030=CARTESIAN_POINT ( 'NONE',  ( 43.00000000000000711, 15.25070940071368497, 139.1143251403882459 ) ) ;
#11035=CARTESIAN_POINT ( 'NONE',  ( 32.39917484285220439, 21.75070940071312364, 139.1143251403882459 ) ) ;
#11044=AXIS2_PLACEMENT_3D ( 'NONE', #6329, #5098, #11022 ) ;
#11047=CARTESIAN_POINT ( 'NONE',  ( 93.56770215592470663, 21.75070940071356418, -33.00000000000012790 ) ) ;
#11052=DIRECTION ( 'NONE',  ( 1.110223024625156540E-15, -1.000000000000000000, 0.000000000000000000 ) ) ;
#11061=ORIENTED_EDGE ( 'NONE', *, *, #2144, .F. ) ;
#11062=VECTOR ( 'NONE', #3441, 1000.000000000000000 ) ;
#11064=EDGE_LOOP ( 'NONE', ( #1924, #5157, #6631, #7960 ) ) ;
#11067=LINE ( 'NONE', #12226, #14577 ) ;
#11070=VECTOR ( 'NONE', #562, 1000.000000000000000 ) ;
#11073=ADVANCED_BREP_SHAPE_REPRESENTATION ( '', ( #8947, #6315 ), #417 ) ;
#11074=ORIENTED_EDGE ( 'NONE', *, *, #4885, .T. ) ;
#11083=ORIENTED_EDGE ( 'NONE', *, *, #6227, .T. ) ;
#11093=ORIENTED_EDGE ( 'NONE', *, *, #2072, .F. ) ;
#11096=DIRECTION ( 'NONE',  ( 1.000000000000000000, 0.000000000000000000, 0.000000000000000000 ) ) ;
#11108=ADVANCED_FACE ( 'NONE', ( #3225 ), #7929, .F. ) ;
#11110=EDGE_LOOP ( 'NONE', ( #6400, #12422, #220, #2821 ) ) ;
#11113=VECTOR ( 'NONE', #5539, 1000.000000000000000 ) ;
#11114=ORIENTED_EDGE ( 'NONE', *, *, #3210, .T. ) ;
#11116=PLANE ( 'NONE',  #7666 ) ;
#11121=EDGE_CURVE ( 'NONE', #6007, #9917, #11611, .T. ) ;
#11122=DIRECTION ( 'NONE',  ( 0.000000000000000000, 1.000000000000000000, -0.000000000000000000 ) ) ;
#11123=VECTOR ( 'NONE', #8355, 1000.000000000000000 ) ;
#11125=CARTESIAN_POINT ( 'NONE',  ( 100.0000000000000284, 0.000000000000000000, 33.00000000000012790 ) ) ;
#11126=LINE ( 'NONE', #1593, #5601 ) ;
#11127=VECTOR ( 'NONE', #7554, 1000.000000000000000 ) ;
#11129=DIRECTION ( 'NONE',  ( 1.000000000000000000, 0.000000000000000000, 0.000000000000000000 ) ) ;
#11131=FACE_OUTER_BOUND ( 'NONE', #1225, .T. ) ;
#11132=VERTEX_POINT ( 'NONE', #8391 ) ;
#11141=VERTEX_POINT ( 'NONE', #2872 ) ;
#11145=EDGE_CURVE ( 'NONE', #6102, #587, #11841, .T. ) ;
#11152=CARTESIAN_POINT ( 'NONE',  ( 112.9262740340969060, 21.75070940071369918, -13.14990448602693007 ) ) ;
#11153=ORIENTED_EDGE ( 'NONE', *, *, #13676, .T. ) ;
#11156=DIRECTION ( 'NONE',  ( 0.000000000000000000, -0.000000000000000000, 1.000000000000000000 ) ) ;
#11160=DIRECTION ( 'NONE',  ( 0.000000000000000000, 1.000000000000000000, -0.000000000000000000 ) ) ;
#11164=FACE_OUTER_BOUND ( 'NONE', #13765, .T. ) ;
#11166=DIRECTION ( 'NONE',  ( 8.673617379884035472E-17, -1.000000000000000000, 0.000000000000000000 ) ) ;
#11167=VERTEX_POINT ( 'NONE', #14236 ) ;
#11170=EDGE_LOOP ( 'NONE', ( #12926, #3150, #12402, #12053 ) ) ;
#11193=DIRECTION ( 'NONE',  ( -1.000000000000000000, 0.000000000000000000, 0.000000000000000000 ) ) ;
#11194=CARTESIAN_POINT ( 'NONE',  ( 58.00000000000000711, -2.249290599286307479, 33.00000000000012790 ) ) ;
#11196=EDGE_CURVE ( 'NONE', #358, #1788, #11688, .T. ) ;
#11198=EDGE_CURVE ( 'NONE', #8798, #1834, #8241, .T. ) ;
#11204=VECTOR ( 'NONE', #3286, 1000.000000000000000 ) ;
#11207=DIRECTION ( 'NONE',  ( 0.000000000000000000, 1.000000000000000000, -0.000000000000000000 ) ) ;
#11218=VECTOR ( 'NONE', #13227, 1000.000000000000000 ) ;
#11219=EDGE_LOOP ( 'NONE', ( #2921, #6819, #6527, #11308 ) ) ;
#11221=ORIENTED_EDGE ( 'NONE', *, *, #9676, .F. ) ;
#11238=VECTOR ( 'NONE', #1397, 1000.000000000000000 ) ;
#11239=CARTESIAN_POINT ( 'NONE',  ( 108.0866310645538562, 21.75070940071366365, 13.14990448602693007 ) ) ;
#11241=VERTEX_POINT ( 'NONE', #3761 ) ;
#11247=VECTOR ( 'NONE', #10336, 1000.000000000000000 ) ;
#11249=DIRECTION ( 'NONE',  ( -0.000000000000000000, -0.000000000000000000, 1.000000000000000000 ) ) ;
#11252=ORIENTED_EDGE ( 'NONE', *, *, #7639, .T. ) ;
#11258=VERTEX_POINT ( 'NONE', #2608 ) ;
#11259=LINE ( 'NONE', #12743, #540 ) ;
#11261=ORIENTED_EDGE ( 'NONE', *, *, #2174, .T. ) ;
#11283=VECTOR ( 'NONE', #3471, 1000.000000000000000 ) ;
#11295=ORIENTED_EDGE ( 'NONE', *, *, #9422, .F. ) ;
#11300=CARTESIAN_POINT ( 'NONE',  ( 27.55953187330915810, 23.25070940071368852, 139.1143251403882459 ) ) ;
#11305=ADVANCED_FACE ( 'NONE', ( #7525 ), #13156, .F. ) ;
#11308=ORIENTED_EDGE ( 'NONE', *, *, #2672, .F. ) ;
#11310=CARTESIAN_POINT ( 'NONE',  ( 0.000000000000000000, 21.75070940071319114, 139.1143251403882459 ) ) ;
#11315=ORIENTED_EDGE ( 'NONE', *, *, #13841, .F. ) ;
#11316=DIRECTION ( 'NONE',  ( -1.000000000000000000, 0.000000000000000000, 0.000000000000000000 ) ) ;
#11326=DIRECTION ( 'NONE',  ( 0.000000000000000000, -0.000000000000000000, 1.000000000000000000 ) ) ;
#11352=DIRECTION ( 'NONE',  ( 0.000000000000000000, 0.000000000000000000, 1.000000000000000000 ) ) ;
#11357=ORIENTED_EDGE ( 'NONE', *, *, #1790, .T. ) ;
#11367=EDGE_CURVE ( 'NONE', #6567, #11241, #3832, .T. ) ;
#11371=ADVANCED_FACE ( 'NONE', ( #6443 ), #13301, .F. ) ;
#11382=PLANE ( 'NONE',  #2423 ) ;
#11388=ADVANCED_FACE ( 'NONE', ( #4047 ), #5293, .F. ) ;
#11390=DIRECTION ( 'NONE',  ( -0.000000000000000000, -0.000000000000000000, -1.000000000000000000 ) ) ;
#11393=CARTESIAN_POINT ( 'NONE',  ( 0.000000000000000000, 2.750709400713692965, 33.00000000000012790 ) ) ;
#11395=CARTESIAN_POINT ( 'NONE',  ( 103.2469880950108063, 0.000000000000000000, -33.00000000000012790 ) ) ;
#11405=ORIENTED_EDGE ( 'NONE', *, *, #15062, .F. ) ;
#11406=DIRECTION ( 'NONE',  ( 1.000000000000000000, 1.156482317317871725E-16, 0.000000000000000000 ) ) ;
#11407=DIRECTION ( 'NONE',  ( 0.000000000000000000, 1.000000000000000000, -0.000000000000000000 ) ) ;
#11409=CARTESIAN_POINT ( 'NONE',  ( 109.8334623555409735, 23.25070940071369563, 33.00000000000012790 ) ) ;
#11413=DIRECTION ( 'NONE',  ( -0.000000000000000000, -0.000000000000000000, -1.000000000000000000 ) ) ;
#11416=LINE ( 'NONE', #12509, #10418 ) ;
#11422=ORIENTED_EDGE ( 'NONE', *, *, #4415, .F. ) ;
#11426=VECTOR ( 'NONE', #5332, 1000.000000000000000 ) ;
#11427=DIRECTION ( 'NONE',  ( -1.000000000000000000, 0.000000000000000000, 0.000000000000000000 ) ) ;
#11439=AXIS2_PLACEMENT_3D ( 'NONE', #3443, #6984, #1120 ) ;
#11440=LINE ( 'NONE', #13916, #5116 ) ;
#11441=ORIENTED_EDGE ( 'NONE', *, *, #8194, .T. ) ;
#11442=CARTESIAN_POINT ( 'NONE',  ( -2.016677571526633510E-15, 23.25070940071368497, 33.00000000000012790 ) ) ;
#11450=CARTESIAN_POINT ( 'NONE',  ( 37.23881781239525424, 0.000000000000000000, -33.00000000000012790 ) ) ;
#11460=ADVANCED_FACE ( 'NONE', ( #7753 ), #5602, .F. ) ;
#11461=VECTOR ( 'NONE', #7194, 1000.000000000000000 ) ;
#11464=ORIENTED_EDGE ( 'NONE', *, *, #13049, .F. ) ;
#11481=ORIENTED_EDGE ( 'NONE', *, *, #14983, .T. ) ;
#11497=CIRCLE ( 'NONE', #4376, 4.000000000000003553 ) ;
#11502=DIRECTION ( 'NONE',  ( -0.000000000000000000, -0.000000000000000000, -1.000000000000000000 ) ) ;
#11505=VERTEX_POINT ( 'NONE', #13752 ) ;
#11515=FACE_OUTER_BOUND ( 'NONE', #14762, .T. ) ;
#11530=ORIENTED_EDGE ( 'NONE', *, *, #4655, .T. ) ;
#11538=LINE ( 'NONE', #9479, #12746 ) ;
#11541=VERTEX_POINT ( 'NONE', #815 ) ;
#11542=DIRECTION ( 'NONE',  ( 1.000000000000000000, 1.110223024625156540E-15, -0.000000000000000000 ) ) ;
#11555=DIRECTION ( 'NONE',  ( -0.000000000000000000, -0.000000000000000000, -1.000000000000000000 ) ) ;
#11561=ORIENTED_EDGE ( 'NONE', *, *, #5470, .F. ) ;
#11563=DIRECTION ( 'NONE',  ( 0.000000000000000000, 1.000000000000000000, 0.000000000000000000 ) ) ;
#11586=DIRECTION ( 'NONE',  ( -0.000000000000000000, -0.000000000000000000, -1.000000000000000000 ) ) ;
#11587=AXIS2_PLACEMENT_3D ( 'NONE', #13772, #12786, #4457 ) ;
#11594=VECTOR ( 'NONE', #2843, 1000.000000000000000 ) ;
#11605=LINE ( 'NONE', #11442, #11113 ) ;
#11606=EDGE_CURVE ( 'NONE', #12694, #12778, #8279, .T. ) ;
#11611=LINE ( 'NONE', #14004, #9508 ) ;
#11614=EDGE_CURVE ( 'NONE', #5061, #3925, #5977, .T. ) ;
#11623=VERTEX_POINT ( 'NONE', #10810 ) ;
#11637=DIRECTION ( 'NONE',  ( -0.000000000000000000, -0.000000000000000000, -1.000000000000000000 ) ) ;
#11639=FACE_OUTER_BOUND ( 'NONE', #456, .T. ) ;
#11647=VERTEX_POINT ( 'NONE', #10103 ) ;
#11651=FACE_OUTER_BOUND ( 'NONE', #11684, .T. ) ;
#11657=CARTESIAN_POINT ( 'NONE',  ( -2.016677571526633510E-15, 23.25070940071368497, -33.00000000000012790 ) ) ;
#11670=VERTEX_POINT ( 'NONE', #12407 ) ;
#11671=DIRECTION ( 'NONE',  ( 1.000000000000000000, 1.156482317317870492E-16, 0.000000000000000000 ) ) ;
#11681=DIRECTION ( 'NONE',  ( 0.000000000000000000, 1.000000000000000000, -0.000000000000000000 ) ) ;
#11683=LINE ( 'NONE', #9157, #4593 ) ;
#11684=EDGE_LOOP ( 'NONE', ( #7353, #10884, #9646, #11811 ) ) ;
#11687=ORIENTED_EDGE ( 'NONE', *, *, #4716, .T. ) ;
#11688=LINE ( 'NONE', #1300, #7050 ) ;
#11690=CARTESIAN_POINT ( 'NONE',  ( 130.4454129427046496, 23.25070940071369563, 13.14990448602692474 ) ) ;
#11692=ORIENTED_EDGE ( 'NONE', *, *, #4119, .T. ) ;
#11694=CARTESIAN_POINT ( 'NONE',  ( 118.0000000000000568, 2.046973701652633381E-13, -13.14990448602693007 ) ) ;
#11711=CARTESIAN_POINT ( 'NONE',  ( 118.0000000000000284, 19.25070940071370273, 139.1143251403882459 ) ) ;
#11739=VECTOR ( 'NONE', #12318, 1000.000000000000000 ) ;
#11744=ORIENTED_EDGE ( 'NONE', *, *, #11145, .T. ) ;
#11745=CARTESIAN_POINT ( 'NONE',  ( 98.40734512546775647, 0.000000000000000000, 33.00000000000012790 ) ) ;
#11746=ORIENTED_EDGE ( 'NONE', *, *, #9136, .F. ) ;
#11755=CARTESIAN_POINT ( 'NONE',  ( 32.39917484285220439, 0.000000000000000000, -33.00000000000012790 ) ) ;
#11758=ORIENTED_EDGE ( 'NONE', *, *, #10001, .T. ) ;
#11765=EDGE_CURVE ( 'NONE', #5614, #9539, #6486, .T. ) ;
#11770=DIRECTION ( 'NONE',  ( 0.000000000000000000, 1.000000000000000000, -0.000000000000000000 ) ) ;
#11779=ORIENTED_EDGE ( 'NONE', *, *, #9981, .T. ) ;
#11782=CIRCLE ( 'NONE', #5148, 4.999999999999997335 ) ;
#11790=FACE_OUTER_BOUND ( 'NONE', #6518, .T. ) ;
#11799=DIRECTION ( 'NONE',  ( -1.000000000000000000, -8.673617379884035472E-17, 0.000000000000000000 ) ) ;
#11805=EDGE_CURVE ( 'NONE', #13383, #14721, #4638, .T. ) ;
#11806=ADVANCED_FACE ( 'NONE', ( #12723 ), #6863, .F. ) ;
#11811=ORIENTED_EDGE ( 'NONE', *, *, #12380, .F. ) ;
#11814=ORIENTED_EDGE ( 'NONE', *, *, #7758, .F. ) ;
#11815=DIRECTION ( 'NONE',  ( 0.000000000000000000, -0.000000000000000000, 1.000000000000000000 ) ) ;
#11817=EDGE_LOOP ( 'NONE', ( #14039, #3079, #10921, #3685 ) ) ;
#11823=EDGE_CURVE ( 'NONE', #7134, #2563, #5801, .T. ) ;
#11841=LINE ( 'NONE', #5781, #12444 ) ;
#11845=VECTOR ( 'NONE', #1074, 1000.000000000000000 ) ;
#11847=PLANE ( 'NONE',  #6434 ) ;
#11852=LINE ( 'NONE', #13248, #3529 ) ;
#11856=VECTOR ( 'NONE', #13803, 1000.000000000000000 ) ;
#11859=AXIS2_PLACEMENT_3D ( 'NONE', #10996, #14313, #14529 ) ;
#11862=ADVANCED_FACE ( 'NONE', ( #15182 ), #3483, .F. ) ;
#11871=CYLINDRICAL_SURFACE ( 'NONE', #703, 4.000000000000003553 ) ;
#11874=CARTESIAN_POINT ( 'NONE',  ( 0.000000000000000000, 21.75070940071359615, 33.00000000000012790 ) ) ;
#11876=EDGE_CURVE ( 'NONE', #7143, #6910, #3326, .T. ) ;
#11878=PLANE ( 'NONE',  #719 ) ;
#11883=ORIENTED_EDGE ( 'NONE', *, *, #13106, .F. ) ;
#11886=CARTESIAN_POINT ( 'NONE',  ( 105.5545870572953930, 15.25070940071369563, 139.1143251403882459 ) ) ;
#11890=DIRECTION ( 'NONE',  ( -0.000000000000000000, -0.000000000000000000, -1.000000000000000000 ) ) ;
#11892=DIRECTION ( 'NONE',  ( 1.000000000000000000, 0.000000000000000000, 0.000000000000000000 ) ) ;
#11896=ORIENTED_EDGE ( 'NONE', *, *, #7826, .F. ) ;
#11903=LINE ( 'NONE', #6066, #15070 ) ;
#11906=EDGE_LOOP ( 'NONE', ( #9056, #1692, #3909, #2613 ) ) ;
#11908=CARTESIAN_POINT ( 'NONE',  ( 0.000000000000000000, 21.75070940071369918, 139.1143251403882459 ) ) ;
#11910=ORIENTED_EDGE ( 'NONE', *, *, #4653, .T. ) ;
#11918=CARTESIAN_POINT ( 'NONE',  ( 112.9262740340969060, 21.75070940071369918, 139.1143251403882459 ) ) ;
#11921=LINE ( 'NONE', #12223, #14713 ) ;
#11927=EDGE_LOOP ( 'NONE', ( #114, #8909, #2602, #6826 ) ) ;
#11928=ORIENTED_EDGE ( 'NONE', *, *, #7824, .T. ) ;
#11929=CARTESIAN_POINT ( 'NONE',  ( 118.0000000000000568, 2.046973701652633381E-13, 139.1143251403882459 ) ) ;
#11931=ORIENTED_EDGE ( 'NONE', *, *, #647, .F. ) ;
#11941=CARTESIAN_POINT ( 'NONE',  ( 54.85055839958032209, 0.000000000000000000, 33.00000000000012790 ) ) ;
#11948=DIRECTION ( 'NONE',  ( 0.000000000000000000, 0.000000000000000000, 1.000000000000000000 ) ) ;
#11950=CARTESIAN_POINT ( 'NONE',  ( 46.91810375148135392, 0.000000000000000000, 139.1143251403882459 ) ) ;
#11958=DIRECTION ( 'NONE',  ( -0.000000000000000000, 0.000000000000000000, -1.000000000000000000 ) ) ;
#11959=EDGE_CURVE ( 'NONE', #4834, #12374, #1324, .T. ) ;
#11964=LINE ( 'NONE', #6055, #13686 ) ;
#11965=ORIENTED_EDGE ( 'NONE', *, *, #1382, .F. ) ;
#11981=ORIENTED_EDGE ( 'NONE', *, *, #8390, .F. ) ;
#11995=ORIENTED_EDGE ( 'NONE', *, *, #3630, .T. ) ;
#12014=DIRECTION ( 'NONE',  ( 1.156482317317870492E-16, -1.000000000000000000, 0.000000000000000000 ) ) ;
#12024=ORIENTED_EDGE ( 'NONE', *, *, #7567, .F. ) ;
#12036=LINE ( 'NONE', #8644, #11070 ) ;
#12041=EDGE_CURVE ( 'NONE', #13017, #4396, #14695, .T. ) ;
#12052=DIRECTION ( 'NONE',  ( -1.000000000000000000, 0.000000000000000000, 0.000000000000000000 ) ) ;
#12053=ORIENTED_EDGE ( 'NONE', *, *, #2967, .F. ) ;
#12077=VECTOR ( 'NONE', #14914, 1000.000000000000000 ) ;
#12083=CARTESIAN_POINT ( 'NONE',  ( 104.9938193859979236, 0.000000000000000000, 33.00000000000012790 ) ) ;
#12104=CARTESIAN_POINT ( 'NONE',  ( -2.016677571526633510E-15, 23.25070940071368497, -33.00000000000012790 ) ) ;
#12108=CARTESIAN_POINT ( 'NONE',  ( 112.9262740340969060, 23.25070940071369563, 33.00000000000012790 ) ) ;
#12110=ORIENTED_EDGE ( 'NONE', *, *, #6340, .T. ) ;
#12116=DIRECTION ( 'NONE',  ( -1.000000000000000000, 0.000000000000000000, 0.000000000000000000 ) ) ;
#12117=VECTOR ( 'NONE', #8457, 1000.000000000000000 ) ;
#12126=LINE ( 'NONE', #1583, #291 ) ;
#12130=DIRECTION ( 'NONE',  ( -0.000000000000000000, -0.000000000000000000, -1.000000000000000000 ) ) ;
#12131=LINE ( 'NONE', #62, #4336 ) ;
#12142=CARTESIAN_POINT ( 'NONE',  ( 54.85055839958032209, 0.000000000000000000, -33.00000000000012790 ) ) ;
#12149=DIRECTION ( 'NONE',  ( 8.673617379884035472E-17, -1.000000000000000000, 0.000000000000000000 ) ) ;
#12152=EDGE_CURVE ( 'NONE', #2314, #6609, #9799, .T. ) ;
#12158=DIRECTION ( 'NONE',  ( -0.000000000000000000, -0.000000000000000000, -1.000000000000000000 ) ) ;
#12165=LINE ( 'NONE', #6183, #665 ) ;
#12170=DIRECTION ( 'NONE',  ( 1.000000000000000000, 0.000000000000000000, 0.000000000000000000 ) ) ;
#12171=EDGE_CURVE ( 'NONE', #14067, #9700, #3155, .T. ) ;
#12176=DIRECTION ( 'NONE',  ( 0.000000000000000000, -0.000000000000000000, -1.000000000000000000 ) ) ;
#12182=CARTESIAN_POINT ( 'NONE',  ( 54.85055839958032209, 23.25070940071368852, 33.00000000000012790 ) ) ;
#12186=ORIENTED_EDGE ( 'NONE', *, *, #9582, .T. ) ;
#12191=ORIENTED_EDGE ( 'NONE', *, *, #11606, .F. ) ;
#12197=EDGE_CURVE ( 'NONE', #14796, #10461, #5706, .T. ) ;
#12199=FACE_OUTER_BOUND ( 'NONE', #12613, .T. ) ;
#12201=DIRECTION ( 'NONE',  ( 1.000000000000000000, 0.000000000000000000, -0.000000000000000000 ) ) ;
#12218=ORIENTED_EDGE ( 'NONE', *, *, #7971, .T. ) ;
#12223=CARTESIAN_POINT ( 'NONE',  ( 58.00000000000000711, 23.25070940071368852, 139.1143251403882459 ) ) ;
#12225=EDGE_CURVE ( 'NONE', #8468, #7944, #12696, .T. ) ;
#12226=CARTESIAN_POINT ( 'NONE',  ( 109.8334623555409735, 23.25070940071369563, 139.1143251403882459 ) ) ;
#12229=CARTESIAN_POINT ( 'NONE',  ( 114.0000000000000284, 15.25070940071369563, 33.00000000000012790 ) ) ;
#12230=EDGE_CURVE ( 'NONE', #8078, #2314, #7855, .T. ) ;
#12241=DIRECTION ( 'NONE',  ( -0.000000000000000000, -0.000000000000000000, -1.000000000000000000 ) ) ;
#12248=VECTOR ( 'NONE', #5903, 1000.000000000000000 ) ;
#12250=LINE ( 'NONE', #7627, #14978 ) ;
#12271=DIRECTION ( 'NONE',  ( -0.000000000000000000, -0.000000000000000000, -1.000000000000000000 ) ) ;
#12275=EDGE_CURVE ( 'NONE', #11141, #5016, #8925, .T. ) ;
#12295=VERTEX_POINT ( 'NONE', #3614 ) ;
#12298=ORIENTED_EDGE ( 'NONE', *, *, #12275, .T. ) ;
#12300=DIRECTION ( 'NONE',  ( 1.000000000000000000, 0.000000000000000000, 0.000000000000000000 ) ) ;
#12308=ORIENTED_EDGE ( 'NONE', *, *, #3608, .F. ) ;
#12318=DIRECTION ( 'NONE',  ( 0.000000000000000000, 1.000000000000000000, -0.000000000000000000 ) ) ;
#12323=VERTEX_POINT ( 'NONE', #4925 ) ;
#12325=PLANE ( 'NONE',  #4122 ) ;
#12327=EDGE_CURVE ( 'NONE', #5697, #1905, #235, .T. ) ;
#12328=AXIS2_PLACEMENT_3D ( 'NONE', #4171, #7877, #13567 ) ;
#12329=CARTESIAN_POINT ( 'NONE',  ( -2.016677571526633510E-15, 23.25070940071368497, 33.00000000000012790 ) ) ;
#12339=EDGE_CURVE ( 'NONE', #8234, #8955, #10548, .T. ) ;
#12346=ORIENTED_EDGE ( 'NONE', *, *, #12275, .F. ) ;
#12352=CARTESIAN_POINT ( 'NONE',  ( 45.17127246049422240, 23.25070940071368852, -33.00000000000012790 ) ) ;
#12356=AXIS2_PLACEMENT_3D ( 'NONE', #13968, #15198, #4651 ) ;
#12358=VECTOR ( 'NONE', #6829, 1000.000000000000000 ) ;
#12359=DIRECTION ( 'NONE',  ( 1.000000000000000000, 0.000000000000000000, 0.000000000000000000 ) ) ;
#12364=LINE ( 'NONE', #8895, #14656 ) ;
#12370=LINE ( 'NONE', #13169, #12687 ) ;
#12372=DIRECTION ( 'NONE',  ( 0.000000000000000000, -0.000000000000000000, 1.000000000000000000 ) ) ;
#12374=VERTEX_POINT ( 'NONE', #14163 ) ;
#12379=EDGE_CURVE ( 'NONE', #65, #4729, #8394, .T. ) ;
#12380=EDGE_CURVE ( 'NONE', #14796, #13684, #7231, .T. ) ;
#12381=LINE ( 'NONE', #4210, #7465 ) ;
#12389=DIRECTION ( 'NONE',  ( 1.000000000000000000, 0.000000000000000000, 0.000000000000000000 ) ) ;
#12396=DIRECTION ( 'NONE',  ( 1.734723475976807292E-15, -1.000000000000000000, 0.000000000000000000 ) ) ;
#12399=ORIENTED_EDGE ( 'NONE', *, *, #222, .F. ) ;
#12400=CARTESIAN_POINT ( 'NONE',  ( 95.31453344691183815, 0.000000000000000000, 139.1143251403882459 ) ) ;
#12402=ORIENTED_EDGE ( 'NONE', *, *, #5099, .F. ) ;
#12407=CARTESIAN_POINT ( 'NONE',  ( 112.9262740340969060, 23.25070940071369563, -13.14990448602692474 ) ) ;
#12415=EDGE_CURVE ( 'NONE', #12323, #7276, #2312, .T. ) ;
#12422=ORIENTED_EDGE ( 'NONE', *, *, #5470, .T. ) ;
#12430=ORIENTED_EDGE ( 'NONE', *, *, #1872, .T. ) ;
#12442=LINE ( 'NONE', #6745, #12833 ) ;
#12444=VECTOR ( 'NONE', #4690, 1000.000000000000000 ) ;
#12445=AXIS2_PLACEMENT_3D ( 'NONE', #9902, #14582, #8881 ) ;
#12447=CARTESIAN_POINT ( 'NONE',  ( 114.6731053250840233, 21.75070940071369918, 13.14990448602693007 ) ) ;
#12451=DIRECTION ( 'NONE',  ( 1.000000000000000000, 0.000000000000000000, 0.000000000000000000 ) ) ;
#12452=VECTOR ( 'NONE', #5926, 1000.000000000000000 ) ;
#12453=ORIENTED_EDGE ( 'NONE', *, *, #12197, .T. ) ;
#12456=VERTEX_POINT ( 'NONE', #9990 ) ;
#12461=PLANE ( 'NONE',  #4231 ) ;
#12466=VERTEX_POINT ( 'NONE', #7528 ) ;
#12468=ORIENTED_EDGE ( 'NONE', *, *, #9435, .T. ) ;
#12479=CARTESIAN_POINT ( 'NONE',  ( 93.56770215592470663, 23.25070940071369208, 33.00000000000012790 ) ) ;
#12480=CARTESIAN_POINT ( 'NONE',  ( 0.000000000000000000, 2.750709400713692965, 139.1143251403882459 ) ) ;
#12481=AXIS2_PLACEMENT_3D ( 'NONE', #13382, #9933, #6459 ) ;
#12484=SHAPE_REPRESENTATION_RELATIONSHIP ( 'NONE' , 'NONE' ,  #13539, #11073 ) ;
#12494=ORIENTED_EDGE ( 'NONE', *, *, #7619, .T. ) ;
#12509=CARTESIAN_POINT ( 'NONE',  ( 18.00000000000001066, 0.000000000000000000, 33.00000000000012790 ) ) ;
#12518=EDGE_LOOP ( 'NONE', ( #12917, #3064, #4989, #4446 ) ) ;
#12530=DIRECTION ( 'NONE',  ( 1.000000000000000000, 0.000000000000000000, 0.000000000000000000 ) ) ;
#12533=CARTESIAN_POINT ( 'NONE',  ( 109.8334623555409735, 0.000000000000000000, -33.00000000000012790 ) ) ;
#12534=ORIENTED_EDGE ( 'NONE', *, *, #6487, .F. ) ;
#12536=DIRECTION ( 'NONE',  ( -0.000000000000000000, -0.000000000000000000, -1.000000000000000000 ) ) ;
#12537=ORIENTED_EDGE ( 'NONE', *, *, #5525, .F. ) ;
#12539=ORIENTED_EDGE ( 'NONE', *, *, #7486, .T. ) ;
#12540=ORIENTED_EDGE ( 'NONE', *, *, #8934, .F. ) ;
#12545=CARTESIAN_POINT ( 'NONE',  ( 112.9262740340969060, 23.25070940071369563, 139.1143251403882459 ) ) ;
#12550=CARTESIAN_POINT ( 'NONE',  ( 118.0000000000000568, 2.046973701652633381E-13, 139.1143251403882459 ) ) ;
#12556=CARTESIAN_POINT ( 'NONE',  ( 58.00000000000000711, 0.000000000000000000, -33.00000000000012790 ) ) ;
#12563=CARTESIAN_POINT ( 'NONE',  ( 0.000000000000000000, 21.75070940071369918, -13.14990448602693007 ) ) ;
#12566=DIRECTION ( 'NONE',  ( -0.000000000000000000, -0.000000000000000000, -1.000000000000000000 ) ) ;
#12578=CARTESIAN_POINT ( 'NONE',  ( 51.75774672102440377, 21.75070940071325865, 139.1143251403882459 ) ) ;
#12593=CARTESIAN_POINT ( 'NONE',  ( 96.00000000000002842, 2.750709400713692965, 139.1143251403882459 ) ) ;
#12596=VECTOR ( 'NONE', #5918, 1000.000000000000000 ) ;
#12597=ORIENTED_EDGE ( 'NONE', *, *, #10748, .F. ) ;
#12612=CARTESIAN_POINT ( 'NONE',  ( 114.6731053250840233, 23.25070940071369563, -33.00000000000012790 ) ) ;
#12613=EDGE_LOOP ( 'NONE', ( #4399, #6335, #6702, #6290 ) ) ;
#12621=EDGE_CURVE ( 'NONE', #77, #1115, #12442, .T. ) ;
#12623=CARTESIAN_POINT ( 'NONE',  ( -2.688903428702175252E-15, 23.25070940071368142, 139.1143251403882459 ) ) ;
#12624=LINE ( 'NONE', #3077, #10890 ) ;
#12633=ORIENTED_EDGE ( 'NONE', *, *, #4576, .T. ) ;
#12634=DIRECTION ( 'NONE',  ( -0.000000000000000000, -0.000000000000000000, -1.000000000000000000 ) ) ;
#12641=PLANE ( 'NONE',  #4736 ) ;
#12653=CARTESIAN_POINT ( 'NONE',  ( 40.33162949095117966, 0.000000000000000000, 139.1143251403882459 ) ) ;
#12659=ADVANCED_FACE ( 'NONE', ( #10971 ), #13351, .T. ) ;
#12669=VERTEX_POINT ( 'NONE', #6565 ) ;
#12675=EDGE_CURVE ( 'NONE', #8736, #4237, #2812, .T. ) ;
#12676=VECTOR ( 'NONE', #255, 1000.000000000000000 ) ;
#12678=CARTESIAN_POINT ( 'NONE',  ( 109.8334623555409735, 0.000000000000000000, -13.14990448602693007 ) ) ;
#12687=VECTOR ( 'NONE', #514, 1000.000000000000000 ) ;
#12690=DIRECTION ( 'NONE',  ( -1.000000000000000000, -1.156482317317870492E-16, 0.000000000000000000 ) ) ;
#12691=ORIENTED_EDGE ( 'NONE', *, *, #10794, .T. ) ;
#12694=VERTEX_POINT ( 'NONE', #10042 ) ;
#12696=LINE ( 'NONE', #12545, #12940 ) ;
#12697=VECTOR ( 'NONE', #3205, 1000.000000000000000 ) ;
#12712=VECTOR ( 'NONE', #191, 1000.000000000000000 ) ;
#12715=CARTESIAN_POINT ( 'NONE',  ( 0.000000000000000000, 21.75070940071312364, 139.1143251403882459 ) ) ;
#12720=DIRECTION ( 'NONE',  ( -1.000000000000000000, 0.000000000000000000, 0.000000000000000000 ) ) ;
#12723=FACE_OUTER_BOUND ( 'NONE', #8150, .T. ) ;
#12724=PLANE ( 'NONE',  #9492 ) ;
#12736=EDGE_CURVE ( 'NONE', #10906, #977, #13283, .T. ) ;
#12738=FACE_OUTER_BOUND ( 'NONE', #12518, .T. ) ;
#12743=CARTESIAN_POINT ( 'NONE',  ( -2.688903428702175252E-15, 23.25070940071368142, -33.00000000000012790 ) ) ;
#12744=PLANE ( 'NONE',  #13447 ) ;
#12746=VECTOR ( 'NONE', #12634, 1000.000000000000000 ) ;
#12749=LINE ( 'NONE', #3192, #5427 ) ;
#12751=VECTOR ( 'NONE', #5753, 1000.000000000000000 ) ;
#12754=ORIENTED_EDGE ( 'NONE', *, *, #7486, .F. ) ;
#12763=LINE ( 'NONE', #14065, #13678 ) ;
#12765=ORIENTED_EDGE ( 'NONE', *, *, #2820, .T. ) ;
#12772=ORIENTED_EDGE ( 'NONE', *, *, #8937, .T. ) ;
#12774=ADVANCED_FACE ( 'NONE', ( #6419 ), #11116, .F. ) ;
#12778=VERTEX_POINT ( 'NONE', #7964 ) ;
#12784=VECTOR ( 'NONE', #278, 1000.000000000000000 ) ;
#12786=DIRECTION ( 'NONE',  ( 0.000000000000000000, 0.000000000000000000, -1.000000000000000000 ) ) ;
#12788=CARTESIAN_POINT ( 'NONE',  ( -1.243300532054838308E-15, 10.75070940071368142, 33.00000000000012790 ) ) ;
#12797=DIRECTION ( 'NONE',  ( -1.000000000000000000, 5.551115123125787632E-16, 0.000000000000000000 ) ) ;
#12803=DIRECTION ( 'NONE',  ( 1.000000000000000000, 0.000000000000000000, 0.000000000000000000 ) ) ;
#12810=EDGE_CURVE ( 'NONE', #11258, #1460, #10429, .T. ) ;
#12824=VECTOR ( 'NONE', #8479, 1000.000000000000000 ) ;
#12830=ORIENTED_EDGE ( 'NONE', *, *, #1361, .T. ) ;
#12833=VECTOR ( 'NONE', #738, 1000.000000000000000 ) ;
#12835=DIRECTION ( 'NONE',  ( 0.000000000000000000, -0.000000000000000000, -1.000000000000000000 ) ) ;
#12845=ORIENTED_EDGE ( 'NONE', *, *, #5525, .T. ) ;
#12851=LINE ( 'NONE', #13910, #12358 ) ;
#12852=EDGE_CURVE ( 'NONE', #6792, #7944, #3104, .T. ) ;
#12861=AXIS2_PLACEMENT_3D ( 'NONE', #9469, #8392, #2541 ) ;
#12864=ORIENTED_EDGE ( 'NONE', *, *, #14768, .F. ) ;
#12870=EDGE_CURVE ( 'NONE', #11623, #8078, #4411, .T. ) ;
#12878=VECTOR ( 'NONE', #5152, 1000.000000000000000 ) ;
#12887=EDGE_CURVE ( 'NONE', #1549, #5437, #2029, .T. ) ;
#12888=CARTESIAN_POINT ( 'NONE',  ( 43.00000000000000711, 10.25070940071368497, 139.1143251403882459 ) ) ;
#12889=VECTOR ( 'NONE', #13585, 1000.000000000000000 ) ;
#12892=CARTESIAN_POINT ( 'NONE',  ( 114.6731053250840233, 0.000000000000000000, 33.00000000000012790 ) ) ;
#12898=CARTESIAN_POINT ( 'NONE',  ( 27.55953187330915810, 23.25070940071368852, 33.00000000000012790 ) ) ;
#12901=CARTESIAN_POINT ( 'NONE',  ( 30.65234355186507997, 23.25070940071368852, -33.00000000000012790 ) ) ;
#12917=ORIENTED_EDGE ( 'NONE', *, *, #1346, .T. ) ;
#12922=ORIENTED_EDGE ( 'NONE', *, *, #13831, .T. ) ;
#12926=ORIENTED_EDGE ( 'NONE', *, *, #9519, .F. ) ;
#12935=CARTESIAN_POINT ( 'NONE',  ( 45.17127246049422240, 0.000000000000000000, 139.1143251403882459 ) ) ;
#12938=DIRECTION ( 'NONE',  ( -1.000000000000000000, 0.000000000000000000, 0.000000000000000000 ) ) ;
#12940=VECTOR ( 'NONE', #2148, 1000.000000000000000 ) ;
#12957=CARTESIAN_POINT ( 'NONE',  ( 93.56770215592470663, 0.000000000000000000, 33.00000000000012790 ) ) ;
#12958=FACE_OUTER_BOUND ( 'NONE', #7616, .T. ) ;
#12964=ADVANCED_FACE ( 'NONE', ( #3571 ), #5814, .T. ) ;
#12965=EDGE_CURVE ( 'NONE', #3666, #9198, #10502, .T. ) ;
#12968=ORIENTED_EDGE ( 'NONE', *, *, #1883, .T. ) ;
#12970=DIRECTION ( 'NONE',  ( -1.000000000000000000, 0.000000000000000000, 0.000000000000000000 ) ) ;
#12973=LINE ( 'NONE', #2426, #9275 ) ;
#12974=VECTOR ( 'NONE', #11413, 1000.000000000000000 ) ;
#12984=AXIS2_PLACEMENT_3D ( 'NONE', #5027, #8418, #7177 ) ;
#12987=EDGE_LOOP ( 'NONE', ( #1448, #8331, #11114, #13027 ) ) ;
#12988=CARTESIAN_POINT ( 'NONE',  ( 0.000000000000000000, 21.75070940071356418, 139.1143251403882459 ) ) ;
#12991=DIRECTION ( 'NONE',  ( 1.156482317317870492E-16, -1.000000000000000000, 0.000000000000000000 ) ) ;
#12997=VECTOR ( 'NONE', #2273, 1000.000000000000000 ) ;
#13003=ORIENTED_EDGE ( 'NONE', *, *, #7106, .F. ) ;
#13004=ORIENTED_EDGE ( 'NONE', *, *, #13643, .F. ) ;
#13017=VERTEX_POINT ( 'NONE', #10728 ) ;
#13020=VERTEX_POINT ( 'NONE', #4882 ) ;
#13025=AXIS2_PLACEMENT_3D ( 'NONE', #10025, #8861, #7638 ) ;
#13027=ORIENTED_EDGE ( 'NONE', *, *, #13743, .T. ) ;
#13030=DIRECTION ( 'NONE',  ( 0.000000000000000000, 0.000000000000000000, 1.000000000000000000 ) ) ;
#13040=LINE ( 'NONE', #116, #2702 ) ;
#13041=ORIENTED_EDGE ( 'NONE', *, *, #8530, .T. ) ;
#13046=STYLED_ITEM('',(#15244),#8947);
#13049=EDGE_CURVE ( 'NONE', #9539, #10074, #10307, .T. ) ;
#13054=VERTEX_POINT ( 'NONE', #1908 ) ;
#13058=CARTESIAN_POINT ( 'NONE',  ( 37.23881781239525424, 21.75070940071315562, -33.00000000000012790 ) ) ;
#13067=DIRECTION ( 'NONE',  ( 0.000000000000000000, 0.000000000000000000, 1.000000000000000000 ) ) ;
#13081=DIRECTION ( 'NONE',  ( -1.000000000000000000, -1.156482317317870492E-16, 0.000000000000000000 ) ) ;
#13082=DIRECTION ( 'NONE',  ( -1.000000000000000000, 0.000000000000000000, 0.000000000000000000 ) ) ;
#13087=CARTESIAN_POINT ( 'NONE',  ( 93.56770215592470663, 0.000000000000000000, -33.00000000000012790 ) ) ;
#13089=ORIENTED_EDGE ( 'NONE', *, *, #5278, .T. ) ;
#13105=LINE ( 'NONE', #2562, #10390 ) ;
#13106=EDGE_CURVE ( 'NONE', #322, #3968, #11605, .T. ) ;
#13113=CIRCLE ( 'NONE', #5237, 4.000000000000003553 ) ;
#13121=LINE ( 'NONE', #9589, #10398 ) ;
#13132=VERTEX_POINT ( 'NONE', #830 ) ;
#13133=DIRECTION ( 'NONE',  ( 1.000000000000000000, 0.000000000000000000, 0.000000000000000000 ) ) ;
#13141=DIRECTION ( 'NONE',  ( 0.000000000000000000, -1.000000000000000000, 0.000000000000000000 ) ) ;
#13146=VERTEX_POINT ( 'NONE', #1983 ) ;
#13148=LINE ( 'NONE', #2600, #9534 ) ;
#13155=ORIENTED_EDGE ( 'NONE', *, *, #3453, .T. ) ;
#13156=PLANE ( 'NONE',  #4077 ) ;
#13161=ORIENTED_EDGE ( 'NONE', *, *, #3102, .T. ) ;
#13162=LINE ( 'NONE', #7309, #13693 ) ;
#13169=CARTESIAN_POINT ( 'NONE',  ( 27.55953187330915810, 0.000000000000000000, -33.00000000000012790 ) ) ;
#13173=EDGE_CURVE ( 'NONE', #8468, #14864, #4290, .T. ) ;
#13177=DIRECTION ( 'NONE',  ( 1.000000000000000000, 1.156482317317870492E-16, 0.000000000000000000 ) ) ;
#13179=EDGE_CURVE ( 'NONE', #6910, #6609, #6916, .T. ) ;
#13180=CARTESIAN_POINT ( 'NONE',  ( 118.0000000000000284, 19.25070940071370273, -33.00000000000012790 ) ) ;
#13189=CARTESIAN_POINT ( 'NONE',  ( 37.23881781239525424, 23.25070940071368852, 139.1143251403882459 ) ) ;
#13198=VECTOR ( 'NONE', #2738, 1000.000000000000000 ) ;
#13199=FACE_OUTER_BOUND ( 'NONE', #14723, .T. ) ;
#13208=ORIENTED_EDGE ( 'NONE', *, *, #1529, .F. ) ;
#13210=VECTOR ( 'NONE', #2801, 1000.000000000000000 ) ;
#13215=DIRECTION ( 'NONE',  ( 1.000000000000000000, 0.000000000000000000, 0.000000000000000000 ) ) ;
#13218=ORIENTED_EDGE ( 'NONE', *, *, #13179, .T. ) ;
#13227=DIRECTION ( 'NONE',  ( -0.000000000000000000, -0.000000000000000000, -1.000000000000000000 ) ) ;
#13232=AXIS2_PLACEMENT_3D ( 'NONE', #7163, #10940, #5013 ) ;
#13235=ORIENTED_EDGE ( 'NONE', *, *, #2460, .T. ) ;
#13239=EDGE_LOOP ( 'NONE', ( #2757, #10633, #7524, #13727 ) ) ;
#13248=CARTESIAN_POINT ( 'NONE',  ( 40.33162949095117966, 21.75070940071319114, 139.1143251403882459 ) ) ;
#13252=DIRECTION ( 'NONE',  ( 1.734723475976807292E-15, -1.000000000000000000, 0.000000000000000000 ) ) ;
#13253=ORIENTED_EDGE ( 'NONE', *, *, #10832, .F. ) ;
#13254=CARTESIAN_POINT ( 'NONE',  ( 56.59738969056744651, 21.75070940071329417, 33.00000000000012790 ) ) ;
#13262=VECTOR ( 'NONE', #2178, 1000.000000000000000 ) ;
#13265=DIRECTION ( 'NONE',  ( -0.000000000000000000, -0.000000000000000000, -1.000000000000000000 ) ) ;
#13273=CIRCLE ( 'NONE', #6150, 4.000000000000003553 ) ;
#13278=EDGE_LOOP ( 'NONE', ( #12597, #766, #1216, #11441 ) ) ;
#13283=LINE ( 'NONE', #5192, #542 ) ;
#13294=DIRECTION ( 'NONE',  ( 0.000000000000000000, -0.000000000000000000, 1.000000000000000000 ) ) ;
#13301=PLANE ( 'NONE',  #8788 ) ;
#13304=ADVANCED_FACE ( 'NONE', ( #11131 ), #13434, .T. ) ;
#13308=VECTOR ( 'NONE', #11555, 1000.000000000000000 ) ;
#13316=ORIENTED_EDGE ( 'NONE', *, *, #4119, .F. ) ;
#13319=ORIENTED_EDGE ( 'NONE', *, *, #5455, .F. ) ;
#13320=VECTOR ( 'NONE', #14318, 1000.000000000000000 ) ;
#13330=DIRECTION ( 'NONE',  ( 1.000000000000000000, 0.000000000000000000, 0.000000000000000000 ) ) ;
#13334=CARTESIAN_POINT ( 'NONE',  ( 114.6731053250840233, 0.000000000000000000, 13.14990448602693007 ) ) ;
#13344=DIRECTION ( 'NONE',  ( 0.000000000000000000, 1.000000000000000000, -0.000000000000000000 ) ) ;
#13350=LINE ( 'NONE', #7503, #3486 ) ;
#13351=PLANE ( 'NONE',  #5450 ) ;
#13354=VERTEX_POINT ( 'NONE', #8599 ) ;
#13356=CARTESIAN_POINT ( 'NONE',  ( 108.0866310645538562, 21.75070940071366365, 33.00000000000012790 ) ) ;
#13358=EDGE_LOOP ( 'NONE', ( #11965, #5075, #2189, #13161 ) ) ;
#13364=DIRECTION ( 'NONE',  ( 0.000000000000000000, 1.000000000000000000, -0.000000000000000000 ) ) ;
#13373=DIRECTION ( 'NONE',  ( 8.673617379884035472E-17, -1.000000000000000000, 0.000000000000000000 ) ) ;
#13379=LINE ( 'NONE', #7610, #4943 ) ;
#13380=LINE ( 'NONE', #7689, #12878 ) ;
#13382=CARTESIAN_POINT ( 'NONE',  ( 0.000000000000000000, 21.75070940071363168, 139.1143251403882459 ) ) ;
#13383=VERTEX_POINT ( 'NONE', #14458 ) ;
#13394=DIRECTION ( 'NONE',  ( 1.000000000000000000, 0.000000000000000000, 0.000000000000000000 ) ) ;
#13397=CARTESIAN_POINT ( 'NONE',  ( 68.00000000000001421, -2.249290599286293268, -33.00000000000012790 ) ) ;
#13400=FACE_OUTER_BOUND ( 'NONE', #2005, .T. ) ;
#13411=VERTEX_POINT ( 'NONE', #10291 ) ;
#13417=CARTESIAN_POINT ( 'NONE',  ( 100.1541764164548880, 21.75070940071359615, 139.1143251403882459 ) ) ;
#13430=CIRCLE ( 'NONE', #4857, 4.000000000000003553 ) ;
#13434=PLANE ( 'NONE',  #3746 ) ;
#13443=DIRECTION ( 'NONE',  ( 1.000000000000000000, 0.000000000000000000, 0.000000000000000000 ) ) ;
#13444=CARTESIAN_POINT ( 'NONE',  ( 48.00000000000000711, 10.25070940071368497, 33.00000000000012790 ) ) ;
#13447=AXIS2_PLACEMENT_3D ( 'NONE', #7968, #1948, #9274 ) ;
#13449=EDGE_CURVE ( 'NONE', #1506, #4084, #4429, .T. ) ;
#13462=FACE_OUTER_BOUND ( 'NONE', #3088, .T. ) ;
#13470=VERTEX_POINT ( 'NONE', #3283 ) ;
#13471=AXIS2_PLACEMENT_3D ( 'NONE', #686, #8850, #11958 ) ;
#13480=ORIENTED_EDGE ( 'NONE', *, *, #9136, .T. ) ;
#13497=ORIENTED_EDGE ( 'NONE', *, *, #9993, .T. ) ;
#13499=CARTESIAN_POINT ( 'NONE',  ( 100.0000000000000284, 6.750709400713692965, 139.1143251403882459 ) ) ;
#13502=AXIS2_PLACEMENT_3D ( 'NONE', #6673, #13837, #12530 ) ;
#13527=DIRECTION ( 'NONE',  ( -1.000000000000000000, 0.000000000000000000, 0.000000000000000000 ) ) ;
#13533=ORIENTED_EDGE ( 'NONE', *, *, #3344, .T. ) ;
#13534=VERTEX_POINT ( 'NONE', #4511 ) ;
#13539=SHAPE_REPRESENTATION ( 'Upper Sharpening Angle Guide Base', ( #6315 ), #417 ) ;
#13543=VERTEX_POINT ( 'NONE', #9215 ) ;
#13547=DIRECTION ( 'NONE',  ( 1.000000000000000000, 8.673617379884035472E-17, 0.000000000000000000 ) ) ;
#13550=AXIS2_PLACEMENT_3D ( 'NONE', #6401, #12176, #7415 ) ;
#13556=LINE ( 'NONE', #2086, #8639 ) ;
#13563=VECTOR ( 'NONE', #13729, 1000.000000000000000 ) ;
#13567=DIRECTION ( 'NONE',  ( 2.775557561562891351E-15, -1.000000000000000000, 0.000000000000000000 ) ) ;
#13569=DIRECTION ( 'NONE',  ( -1.000000000000000000, 0.000000000000000000, 0.000000000000000000 ) ) ;
#13573=DIRECTION ( 'NONE',  ( -1.000000000000000000, -1.156482317317870492E-16, 0.000000000000000000 ) ) ;
#13579=AXIS2_PLACEMENT_3D ( 'NONE', #2668, #7364, #12052 ) ;
#13585=DIRECTION ( 'NONE',  ( -0.000000000000000000, -0.000000000000000000, 1.000000000000000000 ) ) ;
#13593=ORIENTED_EDGE ( 'NONE', *, *, #8646, .T. ) ;
#13598=VECTOR ( 'NONE', #3349, 1000.000000000000000 ) ;
#13601=ORIENTED_EDGE ( 'NONE', *, *, #8397, .T. ) ;
#13610=EDGE_CURVE ( 'NONE', #6567, #3269, #5830, .T. ) ;
#13611=EDGE_CURVE ( 'NONE', #13470, #1907, #8144, .T. ) ;
#13613=VERTEX_POINT ( 'NONE', #2358 ) ;
#13614=ORIENTED_EDGE ( 'NONE', *, *, #8194, .F. ) ;
#13632=LINE ( 'NONE', #11393, #9831 ) ;
#13636=EDGE_CURVE ( 'NONE', #7134, #7276, #6057, .T. ) ;
#13643=EDGE_CURVE ( 'NONE', #11505, #4816, #57, .T. ) ;
#13644=ORIENTED_EDGE ( 'NONE', *, *, #1790, .F. ) ;
#13652=VERTEX_POINT ( 'NONE', #6979 ) ;
#13653=PLANE ( 'NONE',  #12445 ) ;
#13655=ADVANCED_FACE ( 'NONE', ( #5911 ), #9447, .T. ) ;
#13663=ORIENTED_EDGE ( 'NONE', *, *, #14907, .T. ) ;
#13669=VECTOR ( 'NONE', #5292, 1000.000000000000000 ) ;
#13676=EDGE_CURVE ( 'NONE', #9571, #4786, #1275, .T. ) ;
#13678=VECTOR ( 'NONE', #9219, 1000.000000000000000 ) ;
#13682=CARTESIAN_POINT ( 'NONE',  ( 54.85055839958032209, 23.25070940071368852, 139.1143251403882459 ) ) ;
#13684=VERTEX_POINT ( 'NONE', #13058 ) ;
#13686=VECTOR ( 'NONE', #14135, 1000.000000000000000 ) ;
#13688=CARTESIAN_POINT ( 'NONE',  ( -2.688903428702175252E-15, 23.25070940071368142, -33.00000000000012790 ) ) ;
#13691=ORIENTED_EDGE ( 'NONE', *, *, #7824, .F. ) ;
#13693=VECTOR ( 'NONE', #5077, 1000.000000000000000 ) ;
#13701=ORIENTED_EDGE ( 'NONE', *, *, #4799, .F. ) ;
#13703=EDGE_LOOP ( 'NONE', ( #12540, #13593, #10381, #14944 ) ) ;
#13705=LINE ( 'NONE', #7269, #3406 ) ;
#13715=CARTESIAN_POINT ( 'NONE',  ( -2.688903428702175252E-15, 23.25070940071368142, 139.1143251403882459 ) ) ;
#13723=FACE_OUTER_BOUND ( 'NONE', #2117, .T. ) ;
#13727=ORIENTED_EDGE ( 'NONE', *, *, #9981, .F. ) ;
#13729=DIRECTION ( 'NONE',  ( 0.000000000000000000, -1.000000000000000000, 0.000000000000000000 ) ) ;
#13734=EDGE_CURVE ( 'NONE', #13354, #7451, #571, .T. ) ;
#13738=DIRECTION ( 'NONE',  ( 0.000000000000000000, 1.000000000000000000, -0.000000000000000000 ) ) ;
#13739=CARTESIAN_POINT ( 'NONE',  ( 32.39917484285220439, 0.000000000000000000, 33.00000000000012790 ) ) ;
#13742=VERTEX_POINT ( 'NONE', #5191 ) ;
#13743=EDGE_CURVE ( 'NONE', #1788, #1844, #8653, .T. ) ;
#13751=CARTESIAN_POINT ( 'NONE',  ( 95.31453344691183815, 21.75070940071356418, 139.1143251403882459 ) ) ;
#13752=CARTESIAN_POINT ( 'NONE',  ( 98.40734512546775647, 21.75070940071359615, 33.00000000000012790 ) ) ;
#13756=VECTOR ( 'NONE', #7334, 1000.000000000000000 ) ;
#13765=EDGE_LOOP ( 'NONE', ( #3519, #11995, #3703, #1132, #14975, #7693, #3906, #6510, #14063, #8855, #11357, #4585, #365 ) ) ;
#13772=CARTESIAN_POINT ( 'NONE',  ( 96.00000000000002842, 6.750709400713692965, 139.1143251403882459 ) ) ;
#13782=VECTOR ( 'NONE', #11586, 1000.000000000000000 ) ;
#13787=ORIENTED_EDGE ( 'NONE', *, *, #8126, .T. ) ;
#13796=AXIS2_PLACEMENT_3D ( 'NONE', #9343, #2335, #14033 ) ;
#13797=ORIENTED_EDGE ( 'NONE', *, *, #5761, .F. ) ;
#13798=ORIENTED_EDGE ( 'NONE', *, *, #14118, .F. ) ;
#13800=DIRECTION ( 'NONE',  ( 0.000000000000000000, 1.000000000000000000, 0.000000000000000000 ) ) ;
#13803=DIRECTION ( 'NONE',  ( -0.000000000000000000, -0.000000000000000000, -1.000000000000000000 ) ) ;
#13806=DIRECTION ( 'NONE',  ( 0.000000000000000000, 0.000000000000000000, 1.000000000000000000 ) ) ;
#13827=AXIS2_PLACEMENT_3D ( 'NONE', #6121, #1104, #14042 ) ;
#13831=EDGE_CURVE ( 'NONE', #9446, #12466, #13350, .T. ) ;
#13837=DIRECTION ( 'NONE',  ( 0.000000000000000000, -0.000000000000000000, 1.000000000000000000 ) ) ;
#13841=EDGE_CURVE ( 'NONE', #5929, #13543, #12126, .T. ) ;
#13844=ORIENTED_EDGE ( 'NONE', *, *, #8530, .F. ) ;
#13850=FACE_OUTER_BOUND ( 'NONE', #10216, .T. ) ;
#13855=DIRECTION ( 'NONE',  ( -1.000000000000000000, -1.156482317317871725E-16, 0.000000000000000000 ) ) ;
#13856=DIRECTION ( 'NONE',  ( -1.000000000000000000, 0.000000000000000000, 0.000000000000000000 ) ) ;
#13857=FACE_OUTER_BOUND ( 'NONE', #9557, .T. ) ;
#13866=( NAMED_UNIT ( * ) PLANE_ANGLE_UNIT ( ) SI_UNIT ( $, .RADIAN. ) );
#13876=ADVANCED_FACE ( 'NONE', ( #6798 ), #8956, .F. ) ;
#13878=CARTESIAN_POINT ( 'NONE',  ( 32.39917484285220439, 23.25070940071368852, -33.00000000000012790 ) ) ;
#13903=( LENGTH_UNIT ( ) NAMED_UNIT ( * ) SI_UNIT ( .MILLI., .METRE. ) );
#13907=VERTEX_POINT ( 'NONE', #869 ) ;
#13910=CARTESIAN_POINT ( 'NONE',  ( 35.49198652140812982, 21.75070940071315562, 139.1143251403882459 ) ) ;
#13911=EDGE_CURVE ( 'NONE', #15071, #13411, #3266, .T. ) ;
#13916=CARTESIAN_POINT ( 'NONE',  ( 0.000000000000000000, 21.75070940071319114, -33.00000000000012790 ) ) ;
#13918=CARTESIAN_POINT ( 'NONE',  ( 45.17127246049422240, 0.000000000000000000, -33.00000000000012790 ) ) ;
#13927=DIRECTION ( 'NONE',  ( -0.000000000000000000, -0.000000000000000000, -1.000000000000000000 ) ) ;
#13930=ORIENTED_EDGE ( 'NONE', *, *, #7284, .T. ) ;
#13944=PLANE ( 'NONE',  #8587 ) ;
#13966=VECTOR ( 'NONE', #3709, 1000.000000000000000 ) ;
#13968=CARTESIAN_POINT ( 'NONE',  ( 96.00000000000002842, 6.750709400713692965, -33.00000000000014211 ) ) ;
#13983=EDGE_LOOP ( 'NONE', ( #8775, #6286, #13089, #1426 ) ) ;
#13989=ORIENTED_EDGE ( 'NONE', *, *, #8623, .F. ) ;
#13998=DIRECTION ( 'NONE',  ( 1.000000000000000000, 0.000000000000000000, 0.000000000000000000 ) ) ;
#14003=ORIENTED_EDGE ( 'NONE', *, *, #6548, .F. ) ;
#14004=CARTESIAN_POINT ( 'NONE',  ( -2.688903428702175252E-15, 23.25070940071368142, 33.00000000000012790 ) ) ;
#14022=DIRECTION ( 'NONE',  ( -0.000000000000000000, -0.000000000000000000, -1.000000000000000000 ) ) ;
#14027=ADVANCED_FACE ( 'NONE', ( #38 ), #3654, .T. ) ;
#14029=ADVANCED_FACE ( 'NONE', ( #12738 ), #2492, .F. ) ;
#14032=CARTESIAN_POINT ( 'NONE',  ( 37.23881781239525424, 23.25070940071368852, -33.00000000000012790 ) ) ;
#14033=DIRECTION ( 'NONE',  ( 0.000000000000000000, 0.000000000000000000, 1.000000000000000000 ) ) ;
#14038=DIRECTION ( 'NONE',  ( 0.000000000000000000, 0.000000000000000000, 1.000000000000000000 ) ) ;
#14039=ORIENTED_EDGE ( 'NONE', *, *, #3194, .F. ) ;
#14042=DIRECTION ( 'NONE',  ( 0.000000000000000000, -0.000000000000000000, 1.000000000000000000 ) ) ;
#14052=EDGE_CURVE ( 'NONE', #2307, #13742, #5743, .T. ) ;
#14063=ORIENTED_EDGE ( 'NONE', *, *, #12852, .T. ) ;
#14065=CARTESIAN_POINT ( 'NONE',  ( 35.49198652140812982, 23.25070940071368852, 139.1143251403882459 ) ) ;
#14067=VERTEX_POINT ( 'NONE', #12898 ) ;
#14070=VECTOR ( 'NONE', #7807, 1000.000000000000000 ) ;
#14072=DIRECTION ( 'NONE',  ( -1.000000000000000000, 0.000000000000000000, 0.000000000000000000 ) ) ;
#14078=ORIENTED_EDGE ( 'NONE', *, *, #5898, .T. ) ;
#14079=CARTESIAN_POINT ( 'NONE',  ( 0.000000000000000000, 21.75070940071329417, -33.00000000000012790 ) ) ;
#14085=CARTESIAN_POINT ( 'NONE',  ( 43.00000000000000711, 10.25070940071368497, -33.00000000000012790 ) ) ;
#14091=ADVANCED_FACE ( 'NONE', ( #8200 ), #7034, .T. ) ;
#14092=LINE ( 'NONE', #12788, #8771 ) ;
#14095=DIRECTION ( 'NONE',  ( 1.000000000000000000, 0.000000000000000000, 0.000000000000000000 ) ) ;
#14100=ORIENTED_EDGE ( 'NONE', *, *, #6089, .T. ) ;
#14101=FACE_OUTER_BOUND ( 'NONE', #906, .T. ) ;
#14106=ORIENTED_EDGE ( 'NONE', *, *, #7774, .F. ) ;
#14109=PLANE ( 'NONE',  #7379 ) ;
#14113=LINE ( 'NONE', #3565, #13308 ) ;
#14114=EDGE_CURVE ( 'NONE', #8236, #13054, #118, .T. ) ;
#14118=EDGE_CURVE ( 'NONE', #1907, #13470, #4961, .T. ) ;
#14127=ADVANCED_FACE ( 'NONE', ( #8708 ), #8426, .F. ) ;
#14132=DIRECTION ( 'NONE',  ( -1.000000000000000000, -8.673617379884035472E-17, 0.000000000000000000 ) ) ;
#14134=ORIENTED_EDGE ( 'NONE', *, *, #937, .T. ) ;
#14135=DIRECTION ( 'NONE',  ( 0.000000000000000000, 1.000000000000000000, -0.000000000000000000 ) ) ;
#14150=ORIENTED_EDGE ( 'NONE', *, *, #8146, .F. ) ;
#14157=AXIS2_PLACEMENT_3D ( 'NONE', #3250, #9185, #4557 ) ;
#14161=ORIENTED_EDGE ( 'NONE', *, *, #2967, .T. ) ;
#14163=CARTESIAN_POINT ( 'NONE',  ( 118.0000000000000284, 19.25070940071370273, 13.14990448602693007 ) ) ;
#14164=DIRECTION ( 'NONE',  ( 0.000000000000000000, 0.000000000000000000, 1.000000000000000000 ) ) ;
#14174=PLANE ( 'NONE',  #5203 ) ;
#14212=VECTOR ( 'NONE', #10948, 1000.000000000000000 ) ;
#14213=CARTESIAN_POINT ( 'NONE',  ( 114.6731053250840233, 21.75070940071369918, -13.14990448602693007 ) ) ;
#14215=EDGE_CURVE ( 'NONE', #1809, #11258, #9738, .T. ) ;
#14216=CARTESIAN_POINT ( 'NONE',  ( 108.0866310645538562, 0.000000000000000000, 13.14990448602693007 ) ) ;
#14235=VERTEX_POINT ( 'NONE', #6703 ) ;
#14236=CARTESIAN_POINT ( 'NONE',  ( 58.00000000000000711, 10.75070940071368852, 33.00000000000012790 ) ) ;
#14241=VERTEX_POINT ( 'NONE', #12479 ) ;
#14251=FACE_OUTER_BOUND ( 'NONE', #1381, .T. ) ;
#14255=EDGE_LOOP ( 'NONE', ( #8271, #13930, #12968, #7157 ) ) ;
#14257=LINE ( 'NONE', #10638, #11238 ) ;
#14260=PLANE ( 'NONE',  #6874 ) ;
#14266=EDGE_CURVE ( 'NONE', #11670, #8958, #13556, .T. ) ;
#14297=DIRECTION ( 'NONE',  ( -1.000000000000000000, -1.156482317317870492E-16, 0.000000000000000000 ) ) ;
#14301=CARTESIAN_POINT ( 'NONE',  ( 0.000000000000000000, 21.75070940071356418, -33.00000000000012790 ) ) ;
#14302=EDGE_CURVE ( 'NONE', #4834, #358, #5404, .T. ) ;
#14305=ORIENTED_EDGE ( 'NONE', *, *, #4997, .F. ) ;
#14310=ADVANCED_FACE ( 'NONE', ( #14101 ), #5949, .T. ) ;
#14311=VECTOR ( 'NONE', #14546, 1000.000000000000000 ) ;
#14313=DIRECTION ( 'NONE',  ( 0.000000000000000000, 1.000000000000000000, 0.000000000000000000 ) ) ;
#14317=CARTESIAN_POINT ( 'NONE',  ( 108.0866310645538562, 0.000000000000000000, -13.14990448602693007 ) ) ;
#14318=DIRECTION ( 'NONE',  ( -1.734723475976807292E-15, 1.000000000000000000, 0.000000000000000000 ) ) ;
#14338=PLANE ( 'NONE',  #9163 ) ;
#14349=CARTESIAN_POINT ( 'NONE',  ( -2.688903428702175252E-15, 23.25070940071368142, 33.00000000000012790 ) ) ;
#14351=DIRECTION ( 'NONE',  ( -1.000000000000000000, 0.000000000000000000, 0.000000000000000000 ) ) ;
#14355=VECTOR ( 'NONE', #9050, 1000.000000000000000 ) ;
#14360=ADVANCED_FACE ( 'NONE', ( #3553 ), #9481, .F. ) ;
#14365=ORIENTED_EDGE ( 'NONE', *, *, #5054, .T. ) ;
#14370=EDGE_LOOP ( 'NONE', ( #13208, #3442, #4904, #4061 ) ) ;
#14374=ADVANCED_FACE ( 'NONE', ( #4632 ), #14174, .T. ) ;
#14375=CYLINDRICAL_SURFACE ( 'NONE', #13579, 4.000000000000003553 ) ;
#14376=VERTEX_POINT ( 'NONE', #2476 ) ;
#14396=CARTESIAN_POINT ( 'NONE',  ( 56.59738969056744651, 21.75070940071329417, -33.00000000000012790 ) ) ;
#14407=LINE ( 'NONE', #1555, #8550 ) ;
#14413=PLANE ( 'NONE',  #2157 ) ;
#14415=EDGE_CURVE ( 'NONE', #4620, #14067, #3779, .T. ) ;
#14420=LINE ( 'NONE', #13334, #8828 ) ;
#14430=CARTESIAN_POINT ( 'NONE',  ( 58.00000000000000711, -2.249290599286311032, 139.1143251403882459 ) ) ;
#14434=LINE ( 'NONE', #11035, #6151 ) ;
#14436=EDGE_CURVE ( 'NONE', #4285, #12694, #8694, .T. ) ;
#14437=EDGE_LOOP ( 'NONE', ( #6211, #10156, #3842, #4843 ) ) ;
#14439=CARTESIAN_POINT ( 'NONE',  ( -2.688903428702175252E-15, 23.25070940071368142, -33.00000000000012790 ) ) ;
#14440=ORIENTED_EDGE ( 'NONE', *, *, #449, .F. ) ;
#14449=AXIS2_PLACEMENT_3D ( 'NONE', #10551, #6929, #1231 ) ;
#14453=VERTEX_POINT ( 'NONE', #10787 ) ;
#14455=FACE_OUTER_BOUND ( 'NONE', #2883, .T. ) ;
#14457=ORIENTED_EDGE ( 'NONE', *, *, #13179, .F. ) ;
#14458=CARTESIAN_POINT ( 'NONE',  ( 95.31453344691183815, 21.75070940071356418, 33.00000000000012790 ) ) ;
#14480=CARTESIAN_POINT ( 'NONE',  ( 88.00000000000000000, 23.25070940071369208, -33.00000000000012790 ) ) ;
#14485=DIRECTION ( 'NONE',  ( 1.000000000000000000, 0.000000000000000000, 0.000000000000000000 ) ) ;
#14510=DIRECTION ( 'NONE',  ( 0.000000000000000000, 0.000000000000000000, -1.000000000000000000 ) ) ;
#14515=ADVANCED_FACE ( 'NONE', ( #14251 ), #7241, .F. ) ;
#14519=ORIENTED_EDGE ( 'NONE', *, *, #11196, .T. ) ;
#14529=DIRECTION ( 'NONE',  ( 0.000000000000000000, -0.000000000000000000, 1.000000000000000000 ) ) ;
#14530=ORIENTED_EDGE ( 'NONE', *, *, #14215, .F. ) ;
#14538=DIRECTION ( 'NONE',  ( -0.000000000000000000, -0.000000000000000000, -1.000000000000000000 ) ) ;
#14539=ORIENTED_EDGE ( 'NONE', *, *, #15114, .F. ) ;
#14546=DIRECTION ( 'NONE',  ( -0.000000000000000000, -0.000000000000000000, -1.000000000000000000 ) ) ;
#14550=ADVANCED_FACE ( 'NONE', ( #2926 ), #8994, .T. ) ;
#14559=CARTESIAN_POINT ( 'NONE',  ( 25.81270058232203013, 23.25070940071368852, 139.1143251403882459 ) ) ;
#14574=EDGE_LOOP ( 'NONE', ( #5244, #360, #14611, #11692, #8263, #5051, #10275, #14519, #2259, #4983, #8814, #1391, #2904, #4453, #7950, #1047, #7604, #2488, #4609, #3466, #11405, #809, #2328, #2556, #826, #10064, #12430, #13601, #584, #14803, #7764, #8318, #10389, #4191, #3700, #9240, #9717, #14530, #11481, #8673, #13701, #794, #13155, #12765, #529, #729, #3558, #13041, #11561, #7536, #8722, #5193, #14892, #5826, #2680, #12845, #6314, #12754, #11261, #9983, #8018, #10903, #12468, #12308, #589, #14365 ) ) ;
#14576=LINE ( 'NONE', #1581, #2464 ) ;
#14577=VECTOR ( 'NONE', #8913, 1000.000000000000000 ) ;
#14581=LINE ( 'NONE', #6499, #9892 ) ;
#14582=DIRECTION ( 'NONE',  ( -1.000000000000000000, 0.000000000000000000, 0.000000000000000000 ) ) ;
#14598=ORIENTED_EDGE ( 'NONE', *, *, #13676, .F. ) ;
#14611=ORIENTED_EDGE ( 'NONE', *, *, #1382, .T. ) ;
#14628=ORIENTED_EDGE ( 'NONE', *, *, #2260, .F. ) ;
#14643=CARTESIAN_POINT ( 'NONE',  ( 93.56770215592470663, 0.000000000000000000, 139.1143251403882459 ) ) ;
#14644=VERTEX_POINT ( 'NONE', #4063 ) ;
#14656=VECTOR ( 'NONE', #11052, 1000.000000000000000 ) ;
#14658=DIRECTION ( 'NONE',  ( 0.000000000000000000, 0.000000000000000000, 1.000000000000000000 ) ) ;
#14660=ADVANCED_FACE ( 'NONE', ( #13462 ), #3523, .F. ) ;
#14672=ORIENTED_EDGE ( 'NONE', *, *, #12810, .T. ) ;
#14685=CARTESIAN_POINT ( 'NONE',  ( 0.000000000000000000, 21.75070940071309167, 33.00000000000012790 ) ) ;
#14693=CARTESIAN_POINT ( 'NONE',  ( 0.000000000000000000, 21.75070940071329417, 33.00000000000012790 ) ) ;
#14694=VECTOR ( 'NONE', #12451, 1000.000000000000000 ) ;
#14695=LINE ( 'NONE', #5391, #2839 ) ;
#14703=LINE ( 'NONE', #7709, #11127 ) ;
#14704=CARTESIAN_POINT ( 'NONE',  ( 0.000000000000000000, 15.25070940071369563, 33.00000000000012790 ) ) ;
#14708=ORIENTED_EDGE ( 'NONE', *, *, #10748, .T. ) ;
#14713=VECTOR ( 'NONE', #3694, 1000.000000000000000 ) ;
#14720=DIRECTION ( 'NONE',  ( 1.000000000000000000, 0.000000000000000000, 0.000000000000000000 ) ) ;
#14721=VERTEX_POINT ( 'NONE', #575 ) ;
#14723=EDGE_LOOP ( 'NONE', ( #3693, #7048, #10564, #1256 ) ) ;
#14732=EDGE_CURVE ( 'NONE', #10867, #13354, #1807, .T. ) ;
#14738=ORIENTED_EDGE ( 'NONE', *, *, #9756, .T. ) ;
#14760=EDGE_LOOP ( 'NONE', ( #8707, #4703, #12772, #12399 ) ) ;
#14762=EDGE_LOOP ( 'NONE', ( #2682, #6917, #4057, #9845 ) ) ;
#14764=VECTOR ( 'NONE', #1355, 1000.000000000000000 ) ;
#14767=CARTESIAN_POINT ( 'NONE',  ( 88.00000000000001421, 10.75070940071369208, -33.00000000000012790 ) ) ;
#14768=EDGE_CURVE ( 'NONE', #10906, #2535, #14581, .T. ) ;
#14778=EDGE_CURVE ( 'NONE', #13652, #12295, #2881, .T. ) ;
#14782=ADVANCED_FACE ( 'NONE', ( #9753 ), #5274, .F. ) ;
#14783=PLANE ( 'NONE',  #6633 ) ;
#14787=CARTESIAN_POINT ( 'NONE',  ( 130.4454129427046496, 23.25070940071369563, 13.14990448602692474 ) ) ;
#14788=LINE ( 'NONE', #6630, #3253 ) ;
#14792=VECTOR ( 'NONE', #6258, 1000.000000000000000 ) ;
#14796=VERTEX_POINT ( 'NONE', #1511 ) ;
#14803=ORIENTED_EDGE ( 'NONE', *, *, #351, .T. ) ;
#14819=CARTESIAN_POINT ( 'NONE',  ( 114.0000000000000284, 19.25070940071369563, -33.00000000000014211 ) ) ;
#14821=CARTESIAN_POINT ( 'NONE',  ( 109.8334623555409735, 21.75070940071366365, 139.1143251403882459 ) ) ;
#14825=EDGE_CURVE ( 'NONE', #12456, #10618, #7438, .T. ) ;
#14837=CARTESIAN_POINT ( 'NONE',  ( 54.85055839958032209, 21.75070940071329417, 139.1143251403882459 ) ) ;
#14838=ORIENTED_EDGE ( 'NONE', *, *, #3630, .F. ) ;
#14858=ORIENTED_EDGE ( 'NONE', *, *, #2750, .F. ) ;
#14860=FACE_OUTER_BOUND ( 'NONE', #13239, .T. ) ;
#14863=CARTESIAN_POINT ( 'NONE',  ( 27.55953187330915810, 21.75070940071309167, 33.00000000000012790 ) ) ;
#14864=VERTEX_POINT ( 'NONE', #11409 ) ;
#14871=LINE ( 'NONE', #9027, #9634 ) ;
#14885=LINE ( 'NONE', #6730, #12974 ) ;
#14886=DIRECTION ( 'NONE',  ( 0.000000000000000000, 1.000000000000000000, -0.000000000000000000 ) ) ;
#14887=DIRECTION ( 'NONE',  ( -1.000000000000000000, -8.673617379884035472E-17, 0.000000000000000000 ) ) ;
#14892=ORIENTED_EDGE ( 'NONE', *, *, #1361, .F. ) ;
#14902=EDGE_LOOP ( 'NONE', ( #7529, #13480, #7133, #7145 ) ) ;
#14903=VECTOR ( 'NONE', #2815, 1000.000000000000000 ) ;
#14907=EDGE_CURVE ( 'NONE', #13146, #5437, #11259, .T. ) ;
#14914=DIRECTION ( 'NONE',  ( -1.000000000000000000, -1.156482317317870492E-16, 0.000000000000000000 ) ) ;
#14924=DIRECTION ( 'NONE',  ( -0.000000000000000000, -0.000000000000000000, -1.000000000000000000 ) ) ;
#14940=ORIENTED_EDGE ( 'NONE', *, *, #10960, .T. ) ;
#14944=ORIENTED_EDGE ( 'NONE', *, *, #10463, .F. ) ;
#14958=ORIENTED_EDGE ( 'NONE', *, *, #15115, .T. ) ;
#14965=VERTEX_POINT ( 'NONE', #5422 ) ;
#14975=ORIENTED_EDGE ( 'NONE', *, *, #12415, .T. ) ;
#14976=CARTESIAN_POINT ( 'NONE',  ( 93.56770215592470663, 23.25070940071369208, 139.1143251403882459 ) ) ;
#14978=VECTOR ( 'NONE', #7406, 1000.000000000000000 ) ;
#14981=EDGE_LOOP ( 'NONE', ( #871, #12218, #10641, #14106 ) ) ;
#14983=EDGE_CURVE ( 'NONE', #1809, #1117, #4331, .T. ) ;
#14984=CARTESIAN_POINT ( 'NONE',  ( -2.016677571526633510E-15, 23.25070940071368497, 139.1143251403882459 ) ) ;
#14991=LINE ( 'NONE', #2134, #5400 ) ;
#14993=CARTESIAN_POINT ( 'NONE',  ( 56.59738969056744651, 23.25070940071368852, 33.00000000000012790 ) ) ;
#14997=DIRECTION ( 'NONE',  ( 1.000000000000000000, 0.000000000000000000, 0.000000000000000000 ) ) ;
#14999=DIRECTION ( 'NONE',  ( 0.000000000000000000, 1.000000000000000000, -0.000000000000000000 ) ) ;
#15012=FACE_OUTER_BOUND ( 'NONE', #2433, .T. ) ;
#15025=ADVANCED_FACE ( 'NONE', ( #11651 ), #7189, .T. ) ;
#15052=LINE ( 'NONE', #10435, #9372 ) ;
#15060=CIRCLE ( 'NONE', #4016, 4.999999999999997335 ) ;
#15062=EDGE_CURVE ( 'NONE', #12456, #5927, #5973, .T. ) ;
#15067=VECTOR ( 'NONE', #7886, 1000.000000000000000 ) ;
#15070=VECTOR ( 'NONE', #13364, 1000.000000000000000 ) ;
#15071=VERTEX_POINT ( 'NONE', #3572 ) ;
#15074=EDGE_CURVE ( 'NONE', #1691, #65, #120, .T. ) ;
#15081=ORIENTED_EDGE ( 'NONE', *, *, #7776, .F. ) ;
#15083=ORIENTED_EDGE ( 'NONE', *, *, #431, .T. ) ;
#15090=DIRECTION ( 'NONE',  ( 0.000000000000000000, 1.000000000000000000, -0.000000000000000000 ) ) ;
#15093=CARTESIAN_POINT ( 'NONE',  ( 50.01091543003727224, 23.25070940071368852, -33.00000000000012790 ) ) ;
#15105=LINE ( 'NONE', #3323, #8655 ) ;
#15109=PLANE ( 'NONE',  #9878 ) ;
#15114=EDGE_CURVE ( 'NONE', #5252, #1527, #13121, .T. ) ;
#15115=EDGE_CURVE ( 'NONE', #12295, #12778, #3758, .T. ) ;
#15116=VERTEX_POINT ( 'NONE', #12901 ) ;
#15121=ORIENTED_EDGE ( 'NONE', *, *, #7083, .F. ) ;
#15124=DIRECTION ( 'NONE',  ( 1.000000000000000000, 0.000000000000000000, 0.000000000000000000 ) ) ;
#15127=LINE ( 'NONE', #3661, #12751 ) ;
#15131=LINE ( 'NONE', #7823, #916 ) ;
#15153=ORIENTED_EDGE ( 'NONE', *, *, #12379, .F. ) ;
#15163=ADVANCED_FACE ( 'NONE', ( #2425 ), #7264, .T. ) ;
#15169=ORIENTED_EDGE ( 'NONE', *, *, #12225, .T. ) ;
#15170=CARTESIAN_POINT ( 'NONE',  ( 108.0866310645538562, 23.25070940071369563, 13.14990448602692474 ) ) ;
#15181=PRODUCT_DEFINITION_FORMATION_WITH_SPECIFIED_SOURCE ( 'ANY', '', #675, .NOT_KNOWN. ) ;
#15182=FACE_OUTER_BOUND ( 'NONE', #13983, .T. ) ;
#15186=VECTOR ( 'NONE', #1007, 1000.000000000000000 ) ;
#15197=ORIENTED_EDGE ( 'NONE', *, *, #6685, .F. ) ;
#15198=DIRECTION ( 'NONE',  ( 0.000000000000000000, -0.000000000000000000, -1.000000000000000000 ) ) ;
#15213=LINE ( 'NONE', #7903, #2474 ) ;
#15238=COLOUR_RGB('Dark Blue',0.08,0.2,0.34);
#15239=FILL_AREA_STYLE_COLOUR('',#15238);
#15240=FILL_AREA_STYLE('',(#15239));
#15241=SURFACE_STYLE_FILL_AREA(#15240);
#15242=SURFACE_SIDE_STYLE('',(#15241));
#15243=SURFACE_STYLE_USAGE(.BOTH.,#15242);
#15244=PRESENTATION_STYLE_ASSIGNMENT((#15243));
ENDSEC;
END-ISO-10303-21;
